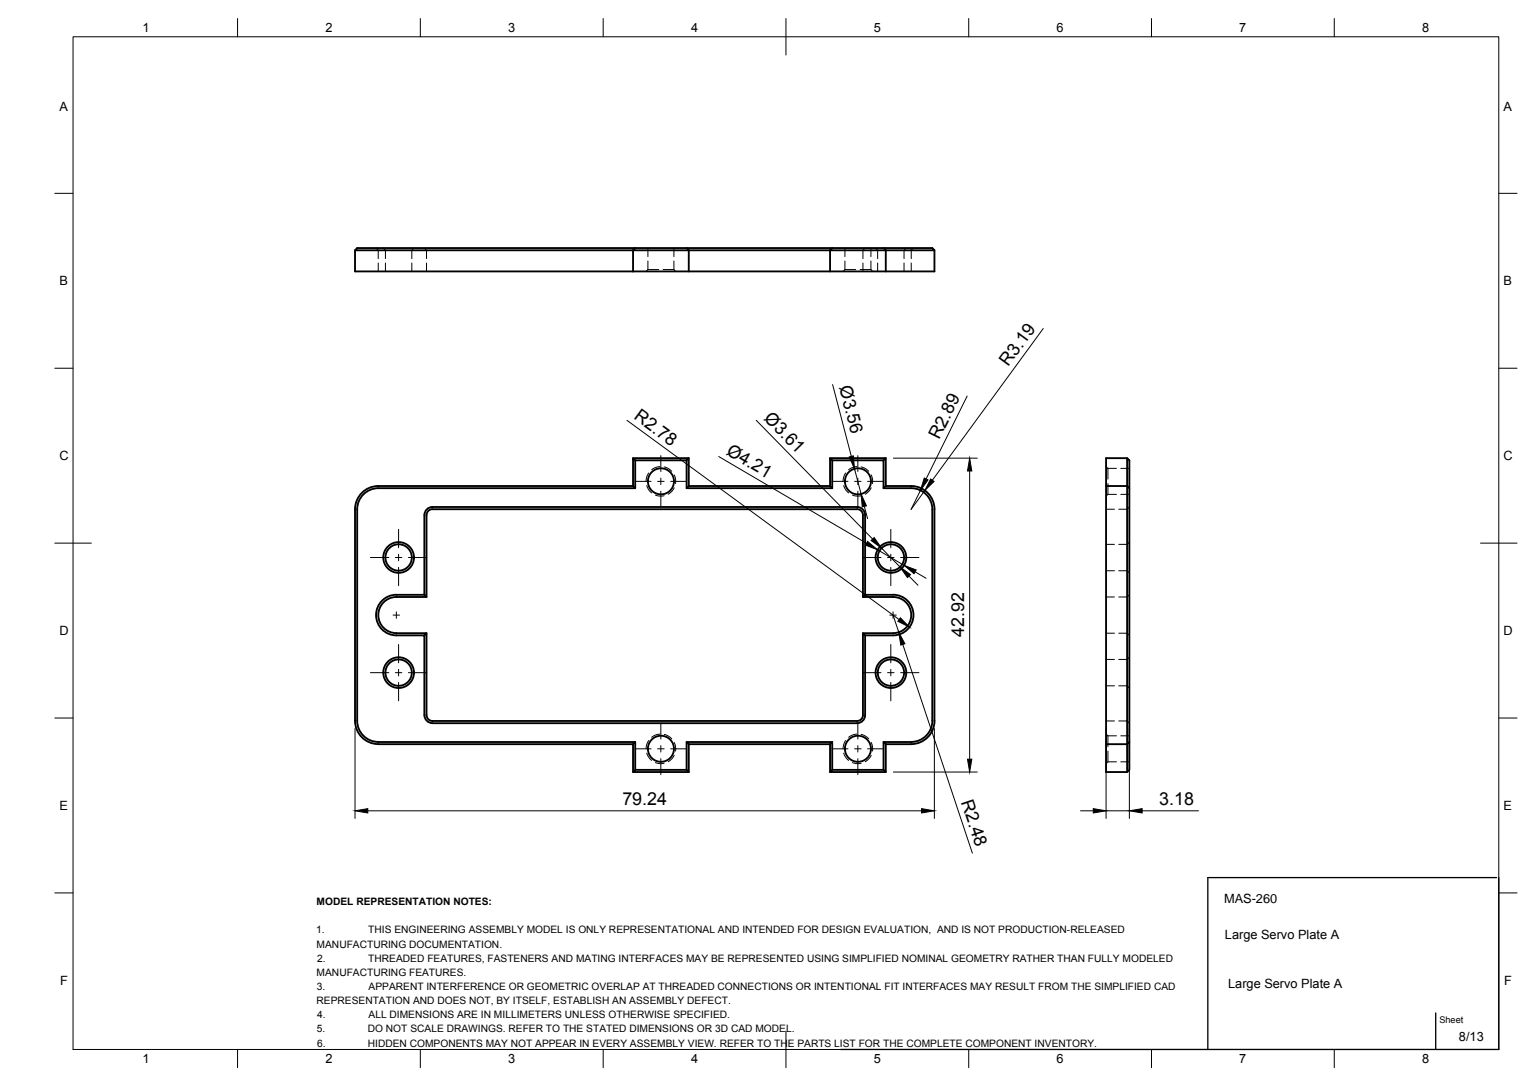
ISO-10303-21;
HEADER;
/* Generated by software containing ST-Developer
 * from STEP Tools, Inc. (www.steptools.com) 
 */

FILE_DESCRIPTION(
/* description */ (''),
/* implementation_level */ '2;1');

FILE_NAME(
/* name */ 'Large Servo Plate A.step',
/* time_stamp */ '2026-10-15T13:29:10-07:00',
/* author */ (''),
/* organization */ (''),
/* preprocessor_version */ 'ST-DEVELOPER v20.2',
/* originating_system */ 'Autodesk Translation Framework v15.15.0.0',
/* authorisation */ '');

FILE_SCHEMA (('AUTOMOTIVE_DESIGN { 1 0 10303 214 3 1 1 }'));
ENDSEC;

DATA;
#10=MECHANICAL_DESIGN_GEOMETRIC_PRESENTATION_REPRESENTATION('',(#934),#83219);
#906=SHAPE_REPRESENTATION_RELATIONSHIP('SRR','None',#83301,#920);
#920=ADVANCED_BREP_SHAPE_REPRESENTATION('',(#948),#83206);
#934=STYLED_ITEM('',(#83380),#948);
#948=MANIFOLD_SOLID_BREP('Body1',#26930);
#983=FACE_BOUND('',#3828,.T.);
#984=FACE_BOUND('',#3829,.T.);
#985=FACE_BOUND('',#3830,.T.);
#986=FACE_BOUND('',#3831,.T.);
#987=FACE_BOUND('',#3832,.T.);
#988=FACE_BOUND('',#3833,.T.);
#989=FACE_BOUND('',#3834,.T.);
#990=FACE_BOUND('',#3835,.T.);
#991=FACE_BOUND('',#3836,.T.);
#992=FACE_BOUND('',#3846,.T.);
#993=FACE_BOUND('',#3847,.T.);
#994=FACE_BOUND('',#3848,.T.);
#995=FACE_BOUND('',#3849,.T.);
#996=FACE_BOUND('',#3850,.T.);
#997=FACE_BOUND('',#3851,.T.);
#998=FACE_BOUND('',#3852,.T.);
#999=FACE_BOUND('',#3853,.T.);
#1000=FACE_BOUND('',#3854,.T.);
#1165=PLANE('',#27211);
#1166=PLANE('',#27246);
#1167=PLANE('',#27270);
#1168=PLANE('',#27271);
#1169=PLANE('',#27272);
#1170=PLANE('',#27273);
#1171=PLANE('',#27274);
#1172=PLANE('',#27275);
#1173=PLANE('',#27276);
#1174=PLANE('',#27277);
#1175=PLANE('',#27278);
#1176=PLANE('',#27279);
#1177=PLANE('',#27280);
#1178=PLANE('',#27281);
#1179=PLANE('',#27282);
#1180=PLANE('',#27285);
#1181=PLANE('',#27288);
#1182=PLANE('',#27291);
#1183=PLANE('',#27294);
#1184=PLANE('',#27295);
#1185=PLANE('',#27296);
#1186=PLANE('',#27297);
#1187=PLANE('',#27298);
#1188=PLANE('',#27299);
#1189=PLANE('',#27300);
#1190=PLANE('',#27301);
#1191=PLANE('',#27302);
#1192=PLANE('',#27303);
#1193=PLANE('',#27304);
#1194=PLANE('',#27305);
#1195=PLANE('',#27307);
#1196=PLANE('',#27309);
#1197=PLANE('',#27310);
#1198=PLANE('',#27311);
#1199=PLANE('',#27312);
#1200=PLANE('',#27315);
#1201=PLANE('',#27316);
#1202=PLANE('',#27319);
#1203=PLANE('',#27322);
#1204=PLANE('',#27325);
#1205=PLANE('',#27328);
#1206=PLANE('',#27331);
#1207=PLANE('',#27332);
#1208=PLANE('',#27334);
#1209=PLANE('',#27335);
#1210=PLANE('',#27337);
#1211=PLANE('',#27339);
#1212=PLANE('',#27340);
#1213=PLANE('',#27341);
#1214=PLANE('',#27343);
#1215=PLANE('',#27344);
#1216=PLANE('',#27346);
#1217=PLANE('',#27348);
#1218=PLANE('',#27349);
#1219=PLANE('',#27350);
#1220=PLANE('',#27351);
#1221=PLANE('',#27352);
#1222=PLANE('',#27353);
#1223=PLANE('',#27354);
#1224=PLANE('',#27355);
#1225=PLANE('',#27357);
#1226=PLANE('',#27359);
#2155=CYLINDRICAL_SURFACE('',#27229,1.778);
#2156=CYLINDRICAL_SURFACE('',#27233,1.778);
#2157=CYLINDRICAL_SURFACE('',#27237,1.778);
#2158=CYLINDRICAL_SURFACE('',#27241,1.778);
#2159=CYLINDRICAL_SURFACE('',#27260,1.8025);
#2160=CYLINDRICAL_SURFACE('',#27263,1.8025);
#2161=CYLINDRICAL_SURFACE('',#27266,1.8025);
#2162=CYLINDRICAL_SURFACE('',#27269,1.8025);
#2163=CYLINDRICAL_SURFACE('',#27306,3.19);
#2164=CYLINDRICAL_SURFACE('',#27308,3.19);
#2165=CYLINDRICAL_SURFACE('',#27333,2.475);
#2166=CYLINDRICAL_SURFACE('',#27336,0.799999999999992);
#2167=CYLINDRICAL_SURFACE('',#27338,0.799999999999994);
#2168=CYLINDRICAL_SURFACE('',#27342,2.475);
#2169=CYLINDRICAL_SURFACE('',#27345,0.799999999999994);
#2170=CYLINDRICAL_SURFACE('',#27347,0.799999999999994);
#2171=CYLINDRICAL_SURFACE('',#27356,3.19);
#2172=CYLINDRICAL_SURFACE('',#27358,3.19);
#2425=FACE_OUTER_BOUND('',#3826,.T.);
#2426=FACE_OUTER_BOUND('',#3827,.T.);
#2427=FACE_OUTER_BOUND('',#3837,.T.);
#2428=FACE_OUTER_BOUND('',#3838,.T.);
#2429=FACE_OUTER_BOUND('',#3839,.T.);
#2430=FACE_OUTER_BOUND('',#3840,.T.);
#2431=FACE_OUTER_BOUND('',#3841,.T.);
#2432=FACE_OUTER_BOUND('',#3842,.T.);
#2433=FACE_OUTER_BOUND('',#3843,.T.);
#2434=FACE_OUTER_BOUND('',#3844,.T.);
#2435=FACE_OUTER_BOUND('',#3845,.T.);
#2436=FACE_OUTER_BOUND('',#3855,.T.);
#2437=FACE_OUTER_BOUND('',#3856,.T.);
#2438=FACE_OUTER_BOUND('',#3857,.T.);
#2439=FACE_OUTER_BOUND('',#3858,.T.);
#2440=FACE_OUTER_BOUND('',#3859,.T.);
#2441=FACE_OUTER_BOUND('',#3860,.T.);
#2442=FACE_OUTER_BOUND('',#3861,.T.);
#2443=FACE_OUTER_BOUND('',#3862,.T.);
#2444=FACE_OUTER_BOUND('',#3863,.T.);
#2445=FACE_OUTER_BOUND('',#3864,.T.);
#2446=FACE_OUTER_BOUND('',#3865,.T.);
#2447=FACE_OUTER_BOUND('',#3866,.T.);
#2448=FACE_OUTER_BOUND('',#3867,.T.);
#2449=FACE_OUTER_BOUND('',#3868,.T.);
#2450=FACE_OUTER_BOUND('',#3869,.T.);
#2451=FACE_OUTER_BOUND('',#3870,.T.);
#2452=FACE_OUTER_BOUND('',#3871,.T.);
#2453=FACE_OUTER_BOUND('',#3872,.T.);
#2454=FACE_OUTER_BOUND('',#3873,.T.);
#2455=FACE_OUTER_BOUND('',#3874,.T.);
#2456=FACE_OUTER_BOUND('',#3875,.T.);
#2457=FACE_OUTER_BOUND('',#3876,.T.);
#2458=FACE_OUTER_BOUND('',#3877,.T.);
#2459=FACE_OUTER_BOUND('',#3878,.T.);
#2460=FACE_OUTER_BOUND('',#3879,.T.);
#2461=FACE_OUTER_BOUND('',#3880,.T.);
#2462=FACE_OUTER_BOUND('',#3881,.T.);
#2463=FACE_OUTER_BOUND('',#3882,.T.);
#2464=FACE_OUTER_BOUND('',#3883,.T.);
#2465=FACE_OUTER_BOUND('',#3884,.T.);
#2466=FACE_OUTER_BOUND('',#3885,.T.);
#2467=FACE_OUTER_BOUND('',#3886,.T.);
#2468=FACE_OUTER_BOUND('',#3887,.T.);
#2469=FACE_OUTER_BOUND('',#3888,.T.);
#2470=FACE_OUTER_BOUND('',#3889,.T.);
#2471=FACE_OUTER_BOUND('',#3890,.T.);
#2472=FACE_OUTER_BOUND('',#3891,.T.);
#2473=FACE_OUTER_BOUND('',#3892,.T.);
#2474=FACE_OUTER_BOUND('',#3893,.T.);
#2475=FACE_OUTER_BOUND('',#3894,.T.);
#2476=FACE_OUTER_BOUND('',#3895,.T.);
#2477=FACE_OUTER_BOUND('',#3896,.T.);
#2478=FACE_OUTER_BOUND('',#3897,.T.);
#2479=FACE_OUTER_BOUND('',#3898,.T.);
#2480=FACE_OUTER_BOUND('',#3899,.T.);
#2481=FACE_OUTER_BOUND('',#3900,.T.);
#2482=FACE_OUTER_BOUND('',#3901,.T.);
#2483=FACE_OUTER_BOUND('',#3902,.T.);
#2484=FACE_OUTER_BOUND('',#3903,.T.);
#2485=FACE_OUTER_BOUND('',#3904,.T.);
#2486=FACE_OUTER_BOUND('',#3905,.T.);
#2487=FACE_OUTER_BOUND('',#3906,.T.);
#2488=FACE_OUTER_BOUND('',#3907,.T.);
#2489=FACE_OUTER_BOUND('',#3908,.T.);
#2490=FACE_OUTER_BOUND('',#3909,.T.);
#2491=FACE_OUTER_BOUND('',#3910,.T.);
#2492=FACE_OUTER_BOUND('',#3911,.T.);
#2493=FACE_OUTER_BOUND('',#3912,.T.);
#2494=FACE_OUTER_BOUND('',#3913,.T.);
#2495=FACE_OUTER_BOUND('',#3914,.T.);
#2496=FACE_OUTER_BOUND('',#3915,.T.);
#2497=FACE_OUTER_BOUND('',#3916,.T.);
#2498=FACE_OUTER_BOUND('',#3917,.T.);
#2499=FACE_OUTER_BOUND('',#3918,.T.);
#2500=FACE_OUTER_BOUND('',#3919,.T.);
#2501=FACE_OUTER_BOUND('',#3920,.T.);
#2502=FACE_OUTER_BOUND('',#3921,.T.);
#2503=FACE_OUTER_BOUND('',#3922,.T.);
#2504=FACE_OUTER_BOUND('',#3923,.T.);
#2505=FACE_OUTER_BOUND('',#3924,.T.);
#2506=FACE_OUTER_BOUND('',#3925,.T.);
#2507=FACE_OUTER_BOUND('',#3926,.T.);
#2508=FACE_OUTER_BOUND('',#3927,.T.);
#2509=FACE_OUTER_BOUND('',#3928,.T.);
#2510=FACE_OUTER_BOUND('',#3929,.T.);
#2511=FACE_OUTER_BOUND('',#3930,.T.);
#2512=FACE_OUTER_BOUND('',#3931,.T.);
#2513=FACE_OUTER_BOUND('',#3932,.T.);
#2514=FACE_OUTER_BOUND('',#3933,.T.);
#2515=FACE_OUTER_BOUND('',#3934,.T.);
#2516=FACE_OUTER_BOUND('',#3935,.T.);
#2517=FACE_OUTER_BOUND('',#3936,.T.);
#2518=FACE_OUTER_BOUND('',#3937,.T.);
#2519=FACE_OUTER_BOUND('',#3938,.T.);
#2520=FACE_OUTER_BOUND('',#3939,.T.);
#2521=FACE_OUTER_BOUND('',#3940,.T.);
#2522=FACE_OUTER_BOUND('',#3941,.T.);
#3826=EDGE_LOOP('',(#17916,#17917,#17918,#17919));
#3827=EDGE_LOOP('',(#17920,#17921,#17922,#17923,#17924,#17925,#17926,#17927,
#17928,#17929,#17930,#17931,#17932,#17933,#17934,#17935,#17936,#17937,#17938,
#17939,#17940,#17941,#17942,#17943));
#3828=EDGE_LOOP('',(#17944));
#3829=EDGE_LOOP('',(#17945));
#3830=EDGE_LOOP('',(#17946));
#3831=EDGE_LOOP('',(#17947));
#3832=EDGE_LOOP('',(#17948));
#3833=EDGE_LOOP('',(#17949));
#3834=EDGE_LOOP('',(#17950,#17951,#17952,#17953,#17954,#17955,#17956,#17957,
#17958,#17959,#17960,#17961,#17962,#17963,#17964,#17965));
#3835=EDGE_LOOP('',(#17966));
#3836=EDGE_LOOP('',(#17967));
#3837=EDGE_LOOP('',(#17968,#17969,#17970,#17971));
#3838=EDGE_LOOP('',(#17972,#17973,#17974,#17975));
#3839=EDGE_LOOP('',(#17976,#17977,#17978,#17979));
#3840=EDGE_LOOP('',(#17980,#17981,#17982,#17983));
#3841=EDGE_LOOP('',(#17984,#17985,#17986,#17987));
#3842=EDGE_LOOP('',(#17988,#17989,#17990,#17991));
#3843=EDGE_LOOP('',(#17992,#17993,#17994,#17995));
#3844=EDGE_LOOP('',(#17996,#17997,#17998,#17999));
#3845=EDGE_LOOP('',(#18000,#18001,#18002,#18003,#18004,#18005,#18006,#18007,
#18008,#18009,#18010,#18011,#18012,#18013,#18014,#18015,#18016,#18017,#18018,
#18019,#18020,#18021,#18022,#18023));
#3846=EDGE_LOOP('',(#18024));
#3847=EDGE_LOOP('',(#18025));
#3848=EDGE_LOOP('',(#18026,#18027,#18028,#18029,#18030,#18031,#18032,#18033,
#18034,#18035,#18036,#18037,#18038,#18039,#18040,#18041));
#3849=EDGE_LOOP('',(#18042));
#3850=EDGE_LOOP('',(#18043));
#3851=EDGE_LOOP('',(#18044));
#3852=EDGE_LOOP('',(#18045));
#3853=EDGE_LOOP('',(#18046));
#3854=EDGE_LOOP('',(#18047));
#3855=EDGE_LOOP('',(#18048,#18049,#18050,#18051));
#3856=EDGE_LOOP('',(#18052,#18053,#18054,#18055));
#3857=EDGE_LOOP('',(#18056,#18057,#18058,#18059));
#3858=EDGE_LOOP('',(#18060,#18061,#18062,#18063));
#3859=EDGE_LOOP('',(#18064,#18065,#18066,#18067));
#3860=EDGE_LOOP('',(#18068,#18069,#18070,#18071));
#3861=EDGE_LOOP('',(#18072,#18073,#18074,#18075));
#3862=EDGE_LOOP('',(#18076,#18077,#18078,#18079));
#3863=EDGE_LOOP('',(#18080,#18081,#18082,#18083));
#3864=EDGE_LOOP('',(#18084,#18085,#18086,#18087));
#3865=EDGE_LOOP('',(#18088,#18089,#18090,#18091));
#3866=EDGE_LOOP('',(#18092,#18093,#18094,#18095));
#3867=EDGE_LOOP('',(#18096,#18097,#18098,#18099));
#3868=EDGE_LOOP('',(#18100,#18101,#18102,#18103));
#3869=EDGE_LOOP('',(#18104,#18105,#18106,#18107));
#3870=EDGE_LOOP('',(#18108,#18109,#18110,#18111));
#3871=EDGE_LOOP('',(#18112,#18113,#18114,#18115));
#3872=EDGE_LOOP('',(#18116,#18117,#18118,#18119));
#3873=EDGE_LOOP('',(#18120,#18121,#18122,#18123));
#3874=EDGE_LOOP('',(#18124,#18125,#18126,#18127));
#3875=EDGE_LOOP('',(#18128,#18129,#18130,#18131));
#3876=EDGE_LOOP('',(#18132,#18133,#18134,#18135));
#3877=EDGE_LOOP('',(#18136,#18137,#18138,#18139));
#3878=EDGE_LOOP('',(#18140,#18141,#18142,#18143));
#3879=EDGE_LOOP('',(#18144,#18145,#18146,#18147));
#3880=EDGE_LOOP('',(#18148,#18149,#18150,#18151));
#3881=EDGE_LOOP('',(#18152,#18153,#18154,#18155));
#3882=EDGE_LOOP('',(#18156,#18157,#18158,#18159));
#3883=EDGE_LOOP('',(#18160,#18161,#18162,#18163));
#3884=EDGE_LOOP('',(#18164,#18165,#18166,#18167));
#3885=EDGE_LOOP('',(#18168,#18169,#18170,#18171));
#3886=EDGE_LOOP('',(#18172,#18173,#18174,#18175));
#3887=EDGE_LOOP('',(#18176,#18177,#18178,#18179));
#3888=EDGE_LOOP('',(#18180,#18181,#18182,#18183));
#3889=EDGE_LOOP('',(#18184,#18185,#18186,#18187));
#3890=EDGE_LOOP('',(#18188,#18189,#18190,#18191));
#3891=EDGE_LOOP('',(#18192,#18193,#18194,#18195));
#3892=EDGE_LOOP('',(#18196,#18197,#18198,#18199));
#3893=EDGE_LOOP('',(#18200,#18201,#18202,#18203));
#3894=EDGE_LOOP('',(#18204,#18205,#18206,#18207));
#3895=EDGE_LOOP('',(#18208,#18209,#18210,#18211));
#3896=EDGE_LOOP('',(#18212,#18213,#18214,#18215));
#3897=EDGE_LOOP('',(#18216,#18217,#18218,#18219));
#3898=EDGE_LOOP('',(#18220,#18221,#18222,#18223));
#3899=EDGE_LOOP('',(#18224,#18225,#18226,#18227));
#3900=EDGE_LOOP('',(#18228,#18229,#18230,#18231));
#3901=EDGE_LOOP('',(#18232,#18233,#18234,#18235));
#3902=EDGE_LOOP('',(#18236,#18237,#18238,#18239));
#3903=EDGE_LOOP('',(#18240,#18241,#18242,#18243));
#3904=EDGE_LOOP('',(#18244,#18245,#18246,#18247));
#3905=EDGE_LOOP('',(#18248,#18249,#18250,#18251));
#3906=EDGE_LOOP('',(#18252,#18253,#18254,#18255));
#3907=EDGE_LOOP('',(#18256,#18257,#18258,#18259));
#3908=EDGE_LOOP('',(#18260,#18261,#18262,#18263));
#3909=EDGE_LOOP('',(#18264,#18265,#18266,#18267));
#3910=EDGE_LOOP('',(#18268,#18269,#18270,#18271));
#3911=EDGE_LOOP('',(#18272,#18273,#18274,#18275));
#3912=EDGE_LOOP('',(#18276,#18277,#18278,#18279));
#3913=EDGE_LOOP('',(#18280,#18281,#18282,#18283));
#3914=EDGE_LOOP('',(#18284,#18285,#18286,#18287));
#3915=EDGE_LOOP('',(#18288,#18289,#18290,#18291));
#3916=EDGE_LOOP('',(#18292,#18293,#18294,#18295));
#3917=EDGE_LOOP('',(#18296,#18297,#18298,#18299));
#3918=EDGE_LOOP('',(#18300,#18301,#18302,#18303));
#3919=EDGE_LOOP('',(#18304,#18305,#18306,#18307));
#3920=EDGE_LOOP('',(#18308,#18309,#18310,#18311));
#3921=EDGE_LOOP('',(#18312,#18313,#18314,#18315));
#3922=EDGE_LOOP('',(#18316,#18317,#18318,#18319));
#3923=EDGE_LOOP('',(#18320,#18321,#18322,#18323));
#3924=EDGE_LOOP('',(#18324,#18325,#18326,#18327));
#3925=EDGE_LOOP('',(#18328,#18329,#18330,#18331));
#3926=EDGE_LOOP('',(#18332,#18333,#18334,#18335));
#3927=EDGE_LOOP('',(#18336,#18337,#18338,#18339));
#3928=EDGE_LOOP('',(#18340,#18341,#18342,#18343));
#3929=EDGE_LOOP('',(#18344,#18345,#18346,#18347));
#3930=EDGE_LOOP('',(#18348,#18349,#18350,#18351));
#3931=EDGE_LOOP('',(#18352,#18353,#18354,#18355));
#3932=EDGE_LOOP('',(#18356,#18357,#18358,#18359));
#3933=EDGE_LOOP('',(#18360,#18361,#18362,#18363));
#3934=EDGE_LOOP('',(#18364,#18365,#18366,#18367));
#3935=EDGE_LOOP('',(#18368,#18369,#18370,#18371));
#3936=EDGE_LOOP('',(#18372,#18373,#18374,#18375));
#3937=EDGE_LOOP('',(#18376,#18377,#18378,#18379));
#3938=EDGE_LOOP('',(#18380,#18381,#18382,#18383));
#3939=EDGE_LOOP('',(#18384,#18385,#18386,#18387));
#3940=EDGE_LOOP('',(#18388,#18389,#18390,#18391));
#3941=EDGE_LOOP('',(#18392,#18393,#18394,#18395));
#5403=LINE('',#36423,#7914);
#5404=LINE('',#36428,#7915);
#5405=LINE('',#36432,#7916);
#5406=LINE('',#36436,#7917);
#5407=LINE('',#36438,#7918);
#5408=LINE('',#36440,#7919);
#5409=LINE('',#36442,#7920);
#5410=LINE('',#36444,#7921);
#5411=LINE('',#36446,#7922);
#5412=LINE('',#36448,#7923);
#5413=LINE('',#36450,#7924);
#5414=LINE('',#36452,#7925);
#5415=LINE('',#36456,#7926);
#5416=LINE('',#36460,#7927);
#5417=LINE('',#36462,#7928);
#5418=LINE('',#36464,#7929);
#5419=LINE('',#36466,#7930);
#5420=LINE('',#36468,#7931);
#5421=LINE('',#36470,#7932);
#5422=LINE('',#36472,#7933);
#5423=LINE('',#36473,#7934);
#5424=LINE('',#36488,#7935);
#5425=LINE('',#36490,#7936);
#5426=LINE('',#36494,#7937);
#5427=LINE('',#36498,#7938);
#5428=LINE('',#36500,#7939);
#5429=LINE('',#36504,#7940);
#5430=LINE('',#36506,#7941);
#5431=LINE('',#36510,#7942);
#5432=LINE('',#36514,#7943);
#5433=LINE('',#36516,#7944);
#5434=LINE('',#36523,#7945);
#5435=LINE('',#36527,#7946);
#5436=LINE('',#36531,#7947);
#5437=LINE('',#36535,#7948);
#5438=LINE('',#36539,#7949);
#5439=LINE('',#36543,#7950);
#5440=LINE('',#36547,#7951);
#5441=LINE('',#36552,#7952);
#5442=LINE('',#36557,#7953);
#5443=LINE('',#36561,#7954);
#5444=LINE('',#36565,#7955);
#5445=LINE('',#36567,#7956);
#5446=LINE('',#36569,#7957);
#5447=LINE('',#36571,#7958);
#5448=LINE('',#36573,#7959);
#5449=LINE('',#36575,#7960);
#5450=LINE('',#36577,#7961);
#5451=LINE('',#36579,#7962);
#5452=LINE('',#36581,#7963);
#5453=LINE('',#36585,#7964);
#5454=LINE('',#36589,#7965);
#5455=LINE('',#36591,#7966);
#5456=LINE('',#36593,#7967);
#5457=LINE('',#36595,#7968);
#5458=LINE('',#36597,#7969);
#5459=LINE('',#36599,#7970);
#5460=LINE('',#36601,#7971);
#5461=LINE('',#36602,#7972);
#5462=LINE('',#36607,#7973);
#5463=LINE('',#36611,#7974);
#5464=LINE('',#36615,#7975);
#5465=LINE('',#36617,#7976);
#5466=LINE('',#36621,#7977);
#5467=LINE('',#36623,#7978);
#5468=LINE('',#36627,#7979);
#5469=LINE('',#36631,#7980);
#5470=LINE('',#36633,#7981);
#5471=LINE('',#36636,#7982);
#5472=LINE('',#36642,#7983);
#5473=LINE('',#36646,#7984);
#5474=LINE('',#36648,#7985);
#5475=LINE('',#36652,#7986);
#5476=LINE('',#36654,#7987);
#5477=LINE('',#36658,#7988);
#5478=LINE('',#36660,#7989);
#5479=LINE('',#36663,#7990);
#5480=LINE('',#36665,#7991);
#5481=LINE('',#36666,#7992);
#5482=LINE('',#36669,#7993);
#5483=LINE('',#36670,#7994);
#5484=LINE('',#36673,#7995);
#5485=LINE('',#36674,#7996);
#5486=LINE('',#36677,#7997);
#5487=LINE('',#36678,#7998);
#5488=LINE('',#36682,#7999);
#5489=LINE('',#36683,#8000);
#5490=LINE('',#36684,#8001);
#5491=LINE('',#36687,#8002);
#5492=LINE('',#36688,#8003);
#5493=LINE('',#36691,#8004);
#5494=LINE('',#36692,#8005);
#5495=LINE('',#36695,#8006);
#5496=LINE('',#36696,#8007);
#5497=LINE('',#36699,#8008);
#5498=LINE('',#36700,#8009);
#5499=LINE('',#36703,#8010);
#5500=LINE('',#36704,#8011);
#5501=LINE('',#36707,#8012);
#5502=LINE('',#36708,#8013);
#5503=LINE('',#36711,#8014);
#5504=LINE('',#36712,#8015);
#5505=LINE('',#36716,#8016);
#5506=LINE('',#36717,#8017);
#5507=LINE('',#36718,#8018);
#5508=LINE('',#36721,#8019);
#5509=LINE('',#36725,#8020);
#5510=LINE('',#36726,#8021);
#5511=LINE('',#36729,#8022);
#5512=LINE('',#36732,#8023);
#5513=LINE('',#36735,#8024);
#5514=LINE('',#36739,#8025);
#5515=LINE('',#36740,#8026);
#5516=LINE('',#36743,#8027);
#5517=LINE('',#36746,#8028);
#5518=LINE('',#36749,#8029);
#5519=LINE('',#36750,#8030);
#5520=LINE('',#36753,#8031);
#5521=LINE('',#36754,#8032);
#5522=LINE('',#36756,#8033);
#5523=LINE('',#36758,#8034);
#5524=LINE('',#36759,#8035);
#5525=LINE('',#36761,#8036);
#5526=LINE('',#36763,#8037);
#5527=LINE('',#36765,#8038);
#5528=LINE('',#36767,#8039);
#5529=LINE('',#36769,#8040);
#5530=LINE('',#36771,#8041);
#5531=LINE('',#36773,#8042);
#5532=LINE('',#36775,#8043);
#5533=LINE('',#36777,#8044);
#5534=LINE('',#36779,#8045);
#5535=LINE('',#36781,#8046);
#5536=LINE('',#36785,#8047);
#5537=LINE('',#36786,#8048);
#5538=LINE('',#36787,#8049);
#5539=LINE('',#36791,#8050);
#5540=LINE('',#36792,#8051);
#5541=LINE('',#36793,#8052);
#5542=LINE('',#36797,#8053);
#5543=LINE('',#36798,#8054);
#5544=LINE('',#36799,#8055);
#5545=LINE('',#36802,#8056);
#5546=LINE('',#36805,#8057);
#5547=LINE('',#36809,#8058);
#5548=LINE('',#36810,#8059);
#5549=LINE('',#36811,#8060);
#5550=LINE('',#36814,#8061);
#5551=LINE('',#36818,#8062);
#5552=LINE('',#36819,#8063);
#5553=LINE('',#36822,#8064);
#5554=LINE('',#36825,#8065);
#5555=LINE('',#36828,#8066);
#5556=LINE('',#36832,#8067);
#5557=LINE('',#36833,#8068);
#5558=LINE('',#36836,#8069);
#5559=LINE('',#36839,#8070);
#5560=LINE('',#36842,#8071);
#5561=LINE('',#36845,#8072);
#5562=LINE('',#36847,#8073);
#5563=LINE('',#36848,#8074);
#5564=LINE('',#36850,#8075);
#5565=LINE('',#36852,#8076);
#5566=LINE('',#36854,#8077);
#5567=LINE('',#36856,#8078);
#5568=LINE('',#36858,#8079);
#5569=LINE('',#36860,#8080);
#5570=LINE('',#36862,#8081);
#5571=LINE('',#36864,#8082);
#5572=LINE('',#36866,#8083);
#5573=LINE('',#36867,#8084);
#5574=LINE('',#36870,#8085);
#5575=LINE('',#36872,#8086);
#5576=LINE('',#36874,#8087);
#5577=LINE('',#36876,#8088);
#5578=LINE('',#36879,#8089);
#5579=LINE('',#36881,#8090);
#5580=LINE('',#36882,#8091);
#5581=LINE('',#36885,#8092);
#5582=LINE('',#36887,#8093);
#5583=LINE('',#36888,#8094);
#5584=LINE('',#36890,#8095);
#5585=LINE('',#36893,#8096);
#5586=LINE('',#36895,#8097);
#5587=LINE('',#36897,#8098);
#5588=LINE('',#36899,#8099);
#7914=VECTOR('',#29605,1.903);
#7915=VECTOR('',#29610,10.);
#7916=VECTOR('',#29613,10.);
#7917=VECTOR('',#29616,10.);
#7918=VECTOR('',#29617,10.);
#7919=VECTOR('',#29618,10.);
#7920=VECTOR('',#29619,10.);
#7921=VECTOR('',#29620,10.);
#7922=VECTOR('',#29621,10.);
#7923=VECTOR('',#29622,10.);
#7924=VECTOR('',#29623,10.);
#7925=VECTOR('',#29624,10.);
#7926=VECTOR('',#29627,10.);
#7927=VECTOR('',#29630,10.);
#7928=VECTOR('',#29631,10.);
#7929=VECTOR('',#29632,10.);
#7930=VECTOR('',#29633,10.);
#7931=VECTOR('',#29634,10.);
#7932=VECTOR('',#29635,10.);
#7933=VECTOR('',#29636,10.);
#7934=VECTOR('',#29637,10.);
#7935=VECTOR('',#29650,10.);
#7936=VECTOR('',#29651,10.);
#7937=VECTOR('',#29654,10.);
#7938=VECTOR('',#29657,10.);
#7939=VECTOR('',#29658,10.);
#7940=VECTOR('',#29661,10.);
#7941=VECTOR('',#29662,10.);
#7942=VECTOR('',#29665,10.);
#7943=VECTOR('',#29668,10.);
#7944=VECTOR('',#29669,10.);
#7945=VECTOR('',#29678,1.778);
#7946=VECTOR('',#29683,1.903);
#7947=VECTOR('',#29688,1.778);
#7948=VECTOR('',#29693,1.903);
#7949=VECTOR('',#29698,1.778);
#7950=VECTOR('',#29703,1.903);
#7951=VECTOR('',#29708,1.778);
#7952=VECTOR('',#29713,1.9525);
#7953=VECTOR('',#29718,10.);
#7954=VECTOR('',#29721,10.);
#7955=VECTOR('',#29724,10.);
#7956=VECTOR('',#29725,10.);
#7957=VECTOR('',#29726,10.);
#7958=VECTOR('',#29727,10.);
#7959=VECTOR('',#29728,10.);
#7960=VECTOR('',#29729,10.);
#7961=VECTOR('',#29730,10.);
#7962=VECTOR('',#29731,10.);
#7963=VECTOR('',#29732,10.);
#7964=VECTOR('',#29735,10.);
#7965=VECTOR('',#29738,10.);
#7966=VECTOR('',#29739,10.);
#7967=VECTOR('',#29740,10.);
#7968=VECTOR('',#29741,10.);
#7969=VECTOR('',#29742,10.);
#7970=VECTOR('',#29743,10.);
#7971=VECTOR('',#29744,10.);
#7972=VECTOR('',#29745,10.);
#7973=VECTOR('',#29748,10.);
#7974=VECTOR('',#29751,10.);
#7975=VECTOR('',#29754,10.);
#7976=VECTOR('',#29755,10.);
#7977=VECTOR('',#29758,10.);
#7978=VECTOR('',#29759,10.);
#7979=VECTOR('',#29762,10.);
#7980=VECTOR('',#29765,10.);
#7981=VECTOR('',#29766,10.);
#7982=VECTOR('',#29769,10.);
#7983=VECTOR('',#29776,1.8025);
#7984=VECTOR('',#29781,1.9525);
#7985=VECTOR('',#29784,1.8025);
#7986=VECTOR('',#29789,1.9525);
#7987=VECTOR('',#29792,1.8025);
#7988=VECTOR('',#29797,1.9525);
#7989=VECTOR('',#29800,1.8025);
#7990=VECTOR('',#29803,10.);
#7991=VECTOR('',#29804,10.);
#7992=VECTOR('',#29805,10.);
#7993=VECTOR('',#29808,10.);
#7994=VECTOR('',#29809,10.);
#7995=VECTOR('',#29812,10.);
#7996=VECTOR('',#29813,10.);
#7997=VECTOR('',#29816,10.);
#7998=VECTOR('',#29817,10.);
#7999=VECTOR('',#29820,10.);
#8000=VECTOR('',#29821,10.);
#8001=VECTOR('',#29822,10.);
#8002=VECTOR('',#29825,10.);
#8003=VECTOR('',#29826,10.);
#8004=VECTOR('',#29829,10.);
#8005=VECTOR('',#29830,10.);
#8006=VECTOR('',#29833,10.);
#8007=VECTOR('',#29834,10.);
#8008=VECTOR('',#29837,10.);
#8009=VECTOR('',#29838,10.);
#8010=VECTOR('',#29841,10.);
#8011=VECTOR('',#29842,10.);
#8012=VECTOR('',#29845,10.);
#8013=VECTOR('',#29846,10.);
#8014=VECTOR('',#29849,10.);
#8015=VECTOR('',#29850,10.);
#8016=VECTOR('',#29853,10.);
#8017=VECTOR('',#29854,10.);
#8018=VECTOR('',#29855,10.);
#8019=VECTOR('',#29858,10.);
#8020=VECTOR('',#29863,10.);
#8021=VECTOR('',#29864,10.);
#8022=VECTOR('',#29867,10.);
#8023=VECTOR('',#29872,10.);
#8024=VECTOR('',#29875,9.99999999999999);
#8025=VECTOR('',#29880,9.99999999999999);
#8026=VECTOR('',#29881,10.);
#8027=VECTOR('',#29884,9.99999999999999);
#8028=VECTOR('',#29889,10.);
#8029=VECTOR('',#29892,10.);
#8030=VECTOR('',#29893,10.);
#8031=VECTOR('',#29896,10.);
#8032=VECTOR('',#29897,10.);
#8033=VECTOR('',#29900,10.);
#8034=VECTOR('',#29903,10.);
#8035=VECTOR('',#29904,10.);
#8036=VECTOR('',#29907,10.);
#8037=VECTOR('',#29910,10.);
#8038=VECTOR('',#29913,10.);
#8039=VECTOR('',#29916,10.);
#8040=VECTOR('',#29919,10.);
#8041=VECTOR('',#29922,10.);
#8042=VECTOR('',#29925,10.);
#8043=VECTOR('',#29928,10.);
#8044=VECTOR('',#29931,10.);
#8045=VECTOR('',#29934,10.);
#8046=VECTOR('',#29937,10.);
#8047=VECTOR('',#29940,10.);
#8048=VECTOR('',#29941,10.);
#8049=VECTOR('',#29942,10.);
#8050=VECTOR('',#29945,10.);
#8051=VECTOR('',#29946,10.);
#8052=VECTOR('',#29947,10.);
#8053=VECTOR('',#29950,10.);
#8054=VECTOR('',#29951,10.);
#8055=VECTOR('',#29952,10.);
#8056=VECTOR('',#29955,10.);
#8057=VECTOR('',#29960,10.);
#8058=VECTOR('',#29963,10.);
#8059=VECTOR('',#29964,10.);
#8060=VECTOR('',#29965,10.);
#8061=VECTOR('',#29968,10.);
#8062=VECTOR('',#29973,10.);
#8063=VECTOR('',#29974,10.);
#8064=VECTOR('',#29977,10.);
#8065=VECTOR('',#29982,10.);
#8066=VECTOR('',#29985,10.);
#8067=VECTOR('',#29990,10.);
#8068=VECTOR('',#29991,10.);
#8069=VECTOR('',#29994,10.);
#8070=VECTOR('',#29999,10.);
#8071=VECTOR('',#30002,9.99999999999999);
#8072=VECTOR('',#30007,10.);
#8073=VECTOR('',#30010,10.);
#8074=VECTOR('',#30011,10.);
#8075=VECTOR('',#30014,10.);
#8076=VECTOR('',#30017,10.);
#8077=VECTOR('',#30020,10.);
#8078=VECTOR('',#30023,10.);
#8079=VECTOR('',#30026,10.);
#8080=VECTOR('',#30029,10.);
#8081=VECTOR('',#30032,10.);
#8082=VECTOR('',#30035,10.);
#8083=VECTOR('',#30038,10.);
#8084=VECTOR('',#30039,10.);
#8085=VECTOR('',#30044,10.);
#8086=VECTOR('',#30047,10.);
#8087=VECTOR('',#30050,10.);
#8088=VECTOR('',#30053,10.);
#8089=VECTOR('',#30058,10.);
#8090=VECTOR('',#30061,10.);
#8091=VECTOR('',#30062,10.);
#8092=VECTOR('',#30067,10.);
#8093=VECTOR('',#30070,10.);
#8094=VECTOR('',#30071,10.);
#8095=VECTOR('',#30074,10.);
#8096=VECTOR('',#30079,10.);
#8097=VECTOR('',#30082,10.);
#8098=VECTOR('',#30085,10.);
#8099=VECTOR('',#30088,10.);
#10338=CIRCLE('',#27209,1.778);
#10339=CIRCLE('',#27210,2.028);
#10340=CIRCLE('',#27212,3.19);
#10341=CIRCLE('',#27213,3.19);
#10342=CIRCLE('',#27214,3.19);
#10343=CIRCLE('',#27215,3.19);
#10344=CIRCLE('',#27216,2.028);
#10345=CIRCLE('',#27217,2.028);
#10346=CIRCLE('',#27218,1.8025);
#10347=CIRCLE('',#27219,1.8025);
#10348=CIRCLE('',#27220,1.8025);
#10349=CIRCLE('',#27221,1.8025);
#10350=CIRCLE('',#27222,0.799999999999992);
#10351=CIRCLE('',#27223,0.799999999999994);
#10352=CIRCLE('',#27224,2.475);
#10353=CIRCLE('',#27225,0.799999999999994);
#10354=CIRCLE('',#27226,0.799999999999994);
#10355=CIRCLE('',#27227,2.475);
#10356=CIRCLE('',#27228,2.028);
#10357=CIRCLE('',#27230,1.778);
#10358=CIRCLE('',#27232,1.778);
#10359=CIRCLE('',#27234,1.778);
#10360=CIRCLE('',#27236,1.778);
#10361=CIRCLE('',#27238,1.778);
#10362=CIRCLE('',#27240,1.778);
#10363=CIRCLE('',#27242,1.778);
#10364=CIRCLE('',#27244,1.8025);
#10365=CIRCLE('',#27245,2.1025);
#10366=CIRCLE('',#27247,2.89);
#10367=CIRCLE('',#27248,2.88999999999999);
#10368=CIRCLE('',#27249,2.89000000000001);
#10369=CIRCLE('',#27250,2.89);
#10370=CIRCLE('',#27251,2.1025);
#10371=CIRCLE('',#27252,1.09999999999999);
#10372=CIRCLE('',#27253,1.1);
#10373=CIRCLE('',#27254,2.775);
#10374=CIRCLE('',#27255,1.1);
#10375=CIRCLE('',#27256,1.09999999999999);
#10376=CIRCLE('',#27257,2.775);
#10377=CIRCLE('',#27258,2.1025);
#10378=CIRCLE('',#27259,2.1025);
#10379=CIRCLE('',#27262,1.8025);
#10380=CIRCLE('',#27265,1.8025);
#10381=CIRCLE('',#27268,1.8025);
#10382=CIRCLE('',#27284,3.19);
#10383=CIRCLE('',#27287,3.19);
#10384=CIRCLE('',#27290,3.19);
#10385=CIRCLE('',#27293,3.19);
#10386=CIRCLE('',#27314,2.475);
#10387=CIRCLE('',#27318,0.799999999999994);
#10388=CIRCLE('',#27321,0.799999999999992);
#10389=CIRCLE('',#27324,0.799999999999994);
#10390=CIRCLE('',#27327,0.799999999999994);
#10391=CIRCLE('',#27330,2.475);
#11154=VERTEX_POINT('',#36420);
#11155=VERTEX_POINT('',#36422);
#11156=VERTEX_POINT('',#36426);
#11157=VERTEX_POINT('',#36427);
#11158=VERTEX_POINT('',#36429);
#11159=VERTEX_POINT('',#36431);
#11160=VERTEX_POINT('',#36433);
#11161=VERTEX_POINT('',#36435);
#11162=VERTEX_POINT('',#36437);
#11163=VERTEX_POINT('',#36439);
#11164=VERTEX_POINT('',#36441);
#11165=VERTEX_POINT('',#36443);
#11166=VERTEX_POINT('',#36445);
#11167=VERTEX_POINT('',#36447);
#11168=VERTEX_POINT('',#36449);
#11169=VERTEX_POINT('',#36451);
#11170=VERTEX_POINT('',#36453);
#11171=VERTEX_POINT('',#36455);
#11172=VERTEX_POINT('',#36457);
#11173=VERTEX_POINT('',#36459);
#11174=VERTEX_POINT('',#36461);
#11175=VERTEX_POINT('',#36463);
#11176=VERTEX_POINT('',#36465);
#11177=VERTEX_POINT('',#36467);
#11178=VERTEX_POINT('',#36469);
#11179=VERTEX_POINT('',#36471);
#11180=VERTEX_POINT('',#36474);
#11181=VERTEX_POINT('',#36476);
#11182=VERTEX_POINT('',#36478);
#11183=VERTEX_POINT('',#36480);
#11184=VERTEX_POINT('',#36482);
#11185=VERTEX_POINT('',#36484);
#11186=VERTEX_POINT('',#36486);
#11187=VERTEX_POINT('',#36487);
#11188=VERTEX_POINT('',#36489);
#11189=VERTEX_POINT('',#36491);
#11190=VERTEX_POINT('',#36493);
#11191=VERTEX_POINT('',#36495);
#11192=VERTEX_POINT('',#36497);
#11193=VERTEX_POINT('',#36499);
#11194=VERTEX_POINT('',#36501);
#11195=VERTEX_POINT('',#36503);
#11196=VERTEX_POINT('',#36505);
#11197=VERTEX_POINT('',#36507);
#11198=VERTEX_POINT('',#36509);
#11199=VERTEX_POINT('',#36511);
#11200=VERTEX_POINT('',#36513);
#11201=VERTEX_POINT('',#36515);
#11202=VERTEX_POINT('',#36518);
#11203=VERTEX_POINT('',#36521);
#11204=VERTEX_POINT('',#36525);
#11205=VERTEX_POINT('',#36529);
#11206=VERTEX_POINT('',#36533);
#11207=VERTEX_POINT('',#36537);
#11208=VERTEX_POINT('',#36541);
#11209=VERTEX_POINT('',#36545);
#11210=VERTEX_POINT('',#36549);
#11211=VERTEX_POINT('',#36551);
#11212=VERTEX_POINT('',#36555);
#11213=VERTEX_POINT('',#36556);
#11214=VERTEX_POINT('',#36558);
#11215=VERTEX_POINT('',#36560);
#11216=VERTEX_POINT('',#36562);
#11217=VERTEX_POINT('',#36564);
#11218=VERTEX_POINT('',#36566);
#11219=VERTEX_POINT('',#36568);
#11220=VERTEX_POINT('',#36570);
#11221=VERTEX_POINT('',#36572);
#11222=VERTEX_POINT('',#36574);
#11223=VERTEX_POINT('',#36576);
#11224=VERTEX_POINT('',#36578);
#11225=VERTEX_POINT('',#36580);
#11226=VERTEX_POINT('',#36582);
#11227=VERTEX_POINT('',#36584);
#11228=VERTEX_POINT('',#36586);
#11229=VERTEX_POINT('',#36588);
#11230=VERTEX_POINT('',#36590);
#11231=VERTEX_POINT('',#36592);
#11232=VERTEX_POINT('',#36594);
#11233=VERTEX_POINT('',#36596);
#11234=VERTEX_POINT('',#36598);
#11235=VERTEX_POINT('',#36600);
#11236=VERTEX_POINT('',#36603);
#11237=VERTEX_POINT('',#36605);
#11238=VERTEX_POINT('',#36606);
#11239=VERTEX_POINT('',#36608);
#11240=VERTEX_POINT('',#36610);
#11241=VERTEX_POINT('',#36612);
#11242=VERTEX_POINT('',#36614);
#11243=VERTEX_POINT('',#36616);
#11244=VERTEX_POINT('',#36618);
#11245=VERTEX_POINT('',#36620);
#11246=VERTEX_POINT('',#36622);
#11247=VERTEX_POINT('',#36624);
#11248=VERTEX_POINT('',#36626);
#11249=VERTEX_POINT('',#36628);
#11250=VERTEX_POINT('',#36630);
#11251=VERTEX_POINT('',#36632);
#11252=VERTEX_POINT('',#36634);
#11253=VERTEX_POINT('',#36637);
#11254=VERTEX_POINT('',#36639);
#11255=VERTEX_POINT('',#36644);
#11256=VERTEX_POINT('',#36650);
#11257=VERTEX_POINT('',#36656);
#11258=VERTEX_POINT('',#36662);
#11259=VERTEX_POINT('',#36664);
#11260=VERTEX_POINT('',#36668);
#11261=VERTEX_POINT('',#36672);
#11262=VERTEX_POINT('',#36676);
#11263=VERTEX_POINT('',#36680);
#11264=VERTEX_POINT('',#36681);
#11265=VERTEX_POINT('',#36686);
#11266=VERTEX_POINT('',#36690);
#11267=VERTEX_POINT('',#36694);
#11268=VERTEX_POINT('',#36698);
#11269=VERTEX_POINT('',#36702);
#11270=VERTEX_POINT('',#36706);
#11271=VERTEX_POINT('',#36710);
#11272=VERTEX_POINT('',#36714);
#11273=VERTEX_POINT('',#36715);
#11274=VERTEX_POINT('',#36720);
#11275=VERTEX_POINT('',#36724);
#11276=VERTEX_POINT('',#36728);
#11277=VERTEX_POINT('',#36734);
#11278=VERTEX_POINT('',#36738);
#11279=VERTEX_POINT('',#36742);
#11280=VERTEX_POINT('',#36748);
#11281=VERTEX_POINT('',#36752);
#11282=VERTEX_POINT('',#36783);
#11283=VERTEX_POINT('',#36784);
#11284=VERTEX_POINT('',#36789);
#11285=VERTEX_POINT('',#36790);
#11286=VERTEX_POINT('',#36795);
#11287=VERTEX_POINT('',#36796);
#11288=VERTEX_POINT('',#36801);
#11289=VERTEX_POINT('',#36807);
#11290=VERTEX_POINT('',#36808);
#11291=VERTEX_POINT('',#36813);
#11292=VERTEX_POINT('',#36817);
#11293=VERTEX_POINT('',#36821);
#11294=VERTEX_POINT('',#36827);
#11295=VERTEX_POINT('',#36831);
#11296=VERTEX_POINT('',#36835);
#11297=VERTEX_POINT('',#36841);
#13819=EDGE_CURVE('',#11154,#11154,#10338,.T.);
#13820=EDGE_CURVE('',#11154,#11155,#5403,.T.);
#13821=EDGE_CURVE('',#11155,#11155,#10339,.T.);
#13822=EDGE_CURVE('',#11156,#11157,#5404,.T.);
#13823=EDGE_CURVE('',#11158,#11157,#10340,.T.);
#13824=EDGE_CURVE('',#11158,#11159,#5405,.T.);
#13825=EDGE_CURVE('',#11160,#11159,#10341,.T.);
#13826=EDGE_CURVE('',#11160,#11161,#5406,.T.);
#13827=EDGE_CURVE('',#11161,#11162,#5407,.T.);
#13828=EDGE_CURVE('',#11162,#11163,#5408,.T.);
#13829=EDGE_CURVE('',#11163,#11164,#5409,.T.);
#13830=EDGE_CURVE('',#11164,#11165,#5410,.T.);
#13831=EDGE_CURVE('',#11165,#11166,#5411,.T.);
#13832=EDGE_CURVE('',#11166,#11167,#5412,.T.);
#13833=EDGE_CURVE('',#11167,#11168,#5413,.T.);
#13834=EDGE_CURVE('',#11168,#11169,#5414,.T.);
#13835=EDGE_CURVE('',#11170,#11169,#10342,.T.);
#13836=EDGE_CURVE('',#11170,#11171,#5415,.T.);
#13837=EDGE_CURVE('',#11172,#11171,#10343,.T.);
#13838=EDGE_CURVE('',#11172,#11173,#5416,.T.);
#13839=EDGE_CURVE('',#11174,#11173,#5417,.T.);
#13840=EDGE_CURVE('',#11175,#11174,#5418,.T.);
#13841=EDGE_CURVE('',#11176,#11175,#5419,.T.);
#13842=EDGE_CURVE('',#11176,#11177,#5420,.T.);
#13843=EDGE_CURVE('',#11178,#11177,#5421,.T.);
#13844=EDGE_CURVE('',#11179,#11178,#5422,.T.);
#13845=EDGE_CURVE('',#11156,#11179,#5423,.T.);
#13846=EDGE_CURVE('',#11180,#11180,#10344,.T.);
#13847=EDGE_CURVE('',#11181,#11181,#10345,.T.);
#13848=EDGE_CURVE('',#11182,#11182,#10346,.T.);
#13849=EDGE_CURVE('',#11183,#11183,#10347,.T.);
#13850=EDGE_CURVE('',#11184,#11184,#10348,.T.);
#13851=EDGE_CURVE('',#11185,#11185,#10349,.T.);
#13852=EDGE_CURVE('',#11186,#11187,#5424,.T.);
#13853=EDGE_CURVE('',#11187,#11188,#5425,.T.);
#13854=EDGE_CURVE('',#11188,#11189,#10350,.T.);
#13855=EDGE_CURVE('',#11189,#11190,#5426,.T.);
#13856=EDGE_CURVE('',#11190,#11191,#10351,.T.);
#13857=EDGE_CURVE('',#11191,#11192,#5427,.T.);
#13858=EDGE_CURVE('',#11192,#11193,#5428,.T.);
#13859=EDGE_CURVE('',#11193,#11194,#10352,.T.);
#13860=EDGE_CURVE('',#11194,#11195,#5429,.T.);
#13861=EDGE_CURVE('',#11195,#11196,#5430,.T.);
#13862=EDGE_CURVE('',#11196,#11197,#10353,.T.);
#13863=EDGE_CURVE('',#11197,#11198,#5431,.T.);
#13864=EDGE_CURVE('',#11198,#11199,#10354,.T.);
#13865=EDGE_CURVE('',#11199,#11200,#5432,.T.);
#13866=EDGE_CURVE('',#11200,#11201,#5433,.T.);
#13867=EDGE_CURVE('',#11201,#11186,#10355,.T.);
#13868=EDGE_CURVE('',#11202,#11202,#10356,.T.);
#13869=EDGE_CURVE('',#11203,#11203,#10357,.T.);
#13870=EDGE_CURVE('',#11203,#11154,#5434,.T.);
#13871=EDGE_CURVE('',#11204,#11204,#10358,.T.);
#13872=EDGE_CURVE('',#11204,#11180,#5435,.T.);
#13873=EDGE_CURVE('',#11205,#11205,#10359,.T.);
#13874=EDGE_CURVE('',#11205,#11204,#5436,.T.);
#13875=EDGE_CURVE('',#11206,#11206,#10360,.T.);
#13876=EDGE_CURVE('',#11206,#11202,#5437,.T.);
#13877=EDGE_CURVE('',#11207,#11207,#10361,.T.);
#13878=EDGE_CURVE('',#11207,#11206,#5438,.T.);
#13879=EDGE_CURVE('',#11208,#11208,#10362,.T.);
#13880=EDGE_CURVE('',#11208,#11181,#5439,.T.);
#13881=EDGE_CURVE('',#11209,#11209,#10363,.T.);
#13882=EDGE_CURVE('',#11209,#11208,#5440,.T.);
#13883=EDGE_CURVE('',#11210,#11210,#10364,.T.);
#13884=EDGE_CURVE('',#11210,#11211,#5441,.T.);
#13885=EDGE_CURVE('',#11211,#11211,#10365,.T.);
#13886=EDGE_CURVE('',#11212,#11213,#5442,.T.);
#13887=EDGE_CURVE('',#11214,#11212,#10366,.T.);
#13888=EDGE_CURVE('',#11215,#11214,#5443,.T.);
#13889=EDGE_CURVE('',#11216,#11215,#10367,.T.);
#13890=EDGE_CURVE('',#11217,#11216,#5444,.T.);
#13891=EDGE_CURVE('',#11218,#11217,#5445,.T.);
#13892=EDGE_CURVE('',#11219,#11218,#5446,.T.);
#13893=EDGE_CURVE('',#11220,#11219,#5447,.T.);
#13894=EDGE_CURVE('',#11221,#11220,#5448,.T.);
#13895=EDGE_CURVE('',#11222,#11221,#5449,.T.);
#13896=EDGE_CURVE('',#11223,#11222,#5450,.T.);
#13897=EDGE_CURVE('',#11224,#11223,#5451,.T.);
#13898=EDGE_CURVE('',#11225,#11224,#5452,.T.);
#13899=EDGE_CURVE('',#11226,#11225,#10368,.T.);
#13900=EDGE_CURVE('',#11227,#11226,#5453,.T.);
#13901=EDGE_CURVE('',#11228,#11227,#10369,.T.);
#13902=EDGE_CURVE('',#11229,#11228,#5454,.T.);
#13903=EDGE_CURVE('',#11230,#11229,#5455,.T.);
#13904=EDGE_CURVE('',#11231,#11230,#5456,.T.);
#13905=EDGE_CURVE('',#11232,#11231,#5457,.T.);
#13906=EDGE_CURVE('',#11233,#11232,#5458,.T.);
#13907=EDGE_CURVE('',#11234,#11233,#5459,.T.);
#13908=EDGE_CURVE('',#11235,#11234,#5460,.T.);
#13909=EDGE_CURVE('',#11213,#11235,#5461,.T.);
#13910=EDGE_CURVE('',#11236,#11236,#10370,.T.);
#13911=EDGE_CURVE('',#11237,#11238,#5462,.T.);
#13912=EDGE_CURVE('',#11239,#11237,#10371,.T.);
#13913=EDGE_CURVE('',#11240,#11239,#5463,.T.);
#13914=EDGE_CURVE('',#11241,#11240,#10372,.T.);
#13915=EDGE_CURVE('',#11242,#11241,#5464,.T.);
#13916=EDGE_CURVE('',#11243,#11242,#5465,.T.);
#13917=EDGE_CURVE('',#11244,#11243,#10373,.T.);
#13918=EDGE_CURVE('',#11245,#11244,#5466,.T.);
#13919=EDGE_CURVE('',#11246,#11245,#5467,.T.);
#13920=EDGE_CURVE('',#11247,#11246,#10374,.T.);
#13921=EDGE_CURVE('',#11248,#11247,#5468,.T.);
#13922=EDGE_CURVE('',#11249,#11248,#10375,.T.);
#13923=EDGE_CURVE('',#11250,#11249,#5469,.T.);
#13924=EDGE_CURVE('',#11251,#11250,#5470,.T.);
#13925=EDGE_CURVE('',#11252,#11251,#10376,.T.);
#13926=EDGE_CURVE('',#11238,#11252,#5471,.T.);
#13927=EDGE_CURVE('',#11253,#11253,#10377,.T.);
#13928=EDGE_CURVE('',#11254,#11254,#10378,.T.);
#13929=EDGE_CURVE('',#11210,#11185,#5472,.T.);
#13930=EDGE_CURVE('',#11255,#11255,#10379,.T.);
#13931=EDGE_CURVE('',#11255,#11254,#5473,.T.);
#13932=EDGE_CURVE('',#11255,#11184,#5474,.T.);
#13933=EDGE_CURVE('',#11256,#11256,#10380,.T.);
#13934=EDGE_CURVE('',#11256,#11236,#5475,.T.);
#13935=EDGE_CURVE('',#11256,#11183,#5476,.T.);
#13936=EDGE_CURVE('',#11257,#11257,#10381,.T.);
#13937=EDGE_CURVE('',#11257,#11253,#5477,.T.);
#13938=EDGE_CURVE('',#11257,#11182,#5478,.T.);
#13939=EDGE_CURVE('',#11232,#11258,#5479,.T.);
#13940=EDGE_CURVE('',#11258,#11259,#5480,.T.);
#13941=EDGE_CURVE('',#11233,#11259,#5481,.T.);
#13942=EDGE_CURVE('',#11231,#11260,#5482,.T.);
#13943=EDGE_CURVE('',#11260,#11258,#5483,.T.);
#13944=EDGE_CURVE('',#11230,#11261,#5484,.T.);
#13945=EDGE_CURVE('',#11261,#11260,#5485,.T.);
#13946=EDGE_CURVE('',#11229,#11262,#5486,.T.);
#13947=EDGE_CURVE('',#11262,#11261,#5487,.T.);
#13948=EDGE_CURVE('',#11263,#11264,#5488,.T.);
#13949=EDGE_CURVE('',#11264,#11225,#5489,.T.);
#13950=EDGE_CURVE('',#11224,#11263,#5490,.T.);
#13951=EDGE_CURVE('',#11223,#11265,#5491,.T.);
#13952=EDGE_CURVE('',#11265,#11263,#5492,.T.);
#13953=EDGE_CURVE('',#11222,#11266,#5493,.T.);
#13954=EDGE_CURVE('',#11266,#11265,#5494,.T.);
#13955=EDGE_CURVE('',#11221,#11267,#5495,.T.);
#13956=EDGE_CURVE('',#11267,#11266,#5496,.T.);
#13957=EDGE_CURVE('',#11220,#11268,#5497,.T.);
#13958=EDGE_CURVE('',#11268,#11267,#5498,.T.);
#13959=EDGE_CURVE('',#11269,#11268,#5499,.T.);
#13960=EDGE_CURVE('',#11219,#11269,#5500,.T.);
#13961=EDGE_CURVE('',#11270,#11269,#5501,.T.);
#13962=EDGE_CURVE('',#11218,#11270,#5502,.T.);
#13963=EDGE_CURVE('',#11271,#11270,#5503,.T.);
#13964=EDGE_CURVE('',#11217,#11271,#5504,.T.);
#13965=EDGE_CURVE('',#11272,#11273,#5505,.T.);
#13966=EDGE_CURVE('',#11273,#11212,#5506,.T.);
#13967=EDGE_CURVE('',#11213,#11272,#5507,.T.);
#13968=EDGE_CURVE('',#11274,#11214,#5508,.T.);
#13969=EDGE_CURVE('',#11273,#11274,#10382,.T.);
#13970=EDGE_CURVE('',#11275,#11215,#5509,.T.);
#13971=EDGE_CURVE('',#11274,#11275,#5510,.T.);
#13972=EDGE_CURVE('',#11276,#11216,#5511,.T.);
#13973=EDGE_CURVE('',#11275,#11276,#10383,.T.);
#13974=EDGE_CURVE('',#11276,#11271,#5512,.T.);
#13975=EDGE_CURVE('',#11277,#11226,#5513,.T.);
#13976=EDGE_CURVE('',#11264,#11277,#10384,.T.);
#13977=EDGE_CURVE('',#11278,#11227,#5514,.T.);
#13978=EDGE_CURVE('',#11277,#11278,#5515,.T.);
#13979=EDGE_CURVE('',#11279,#11228,#5516,.T.);
#13980=EDGE_CURVE('',#11278,#11279,#10385,.T.);
#13981=EDGE_CURVE('',#11279,#11262,#5517,.T.);
#13982=EDGE_CURVE('',#11280,#11272,#5518,.T.);
#13983=EDGE_CURVE('',#11235,#11280,#5519,.T.);
#13984=EDGE_CURVE('',#11281,#11280,#5520,.T.);
#13985=EDGE_CURVE('',#11234,#11281,#5521,.T.);
#13986=EDGE_CURVE('',#11259,#11281,#5522,.T.);
#13987=EDGE_CURVE('',#11174,#11265,#5523,.T.);
#13988=EDGE_CURVE('',#11263,#11173,#5524,.T.);
#13989=EDGE_CURVE('',#11175,#11266,#5525,.T.);
#13990=EDGE_CURVE('',#11176,#11267,#5526,.T.);
#13991=EDGE_CURVE('',#11268,#11177,#5527,.T.);
#13992=EDGE_CURVE('',#11178,#11269,#5528,.T.);
#13993=EDGE_CURVE('',#11179,#11270,#5529,.T.);
#13994=EDGE_CURVE('',#11156,#11271,#5530,.T.);
#13995=EDGE_CURVE('',#11157,#11276,#5531,.T.);
#13996=EDGE_CURVE('',#11158,#11275,#5532,.T.);
#13997=EDGE_CURVE('',#11159,#11274,#5533,.T.);
#13998=EDGE_CURVE('',#11160,#11273,#5534,.T.);
#13999=EDGE_CURVE('',#11272,#11161,#5535,.T.);
#14000=EDGE_CURVE('',#11282,#11283,#5536,.T.);
#14001=EDGE_CURVE('',#11283,#11251,#5537,.T.);
#14002=EDGE_CURVE('',#11250,#11282,#5538,.T.);
#14003=EDGE_CURVE('',#11284,#11285,#5539,.T.);
#14004=EDGE_CURVE('',#11285,#11246,#5540,.T.);
#14005=EDGE_CURVE('',#11245,#11284,#5541,.T.);
#14006=EDGE_CURVE('',#11286,#11287,#5542,.T.);
#14007=EDGE_CURVE('',#11287,#11243,#5543,.T.);
#14008=EDGE_CURVE('',#11242,#11286,#5544,.T.);
#14009=EDGE_CURVE('',#11288,#11244,#5545,.T.);
#14010=EDGE_CURVE('',#11287,#11288,#10386,.T.);
#14011=EDGE_CURVE('',#11288,#11284,#5546,.T.);
#14012=EDGE_CURVE('',#11289,#11290,#5547,.T.);
#14013=EDGE_CURVE('',#11290,#11237,#5548,.T.);
#14014=EDGE_CURVE('',#11238,#11289,#5549,.T.);
#14015=EDGE_CURVE('',#11291,#11239,#5550,.T.);
#14016=EDGE_CURVE('',#11290,#11291,#10387,.T.);
#14017=EDGE_CURVE('',#11292,#11240,#5551,.T.);
#14018=EDGE_CURVE('',#11291,#11292,#5552,.T.);
#14019=EDGE_CURVE('',#11293,#11241,#5553,.T.);
#14020=EDGE_CURVE('',#11292,#11293,#10388,.T.);
#14021=EDGE_CURVE('',#11293,#11286,#5554,.T.);
#14022=EDGE_CURVE('',#11294,#11247,#5555,.T.);
#14023=EDGE_CURVE('',#11285,#11294,#10389,.T.);
#14024=EDGE_CURVE('',#11295,#11248,#5556,.T.);
#14025=EDGE_CURVE('',#11294,#11295,#5557,.T.);
#14026=EDGE_CURVE('',#11296,#11249,#5558,.T.);
#14027=EDGE_CURVE('',#11295,#11296,#10390,.T.);
#14028=EDGE_CURVE('',#11296,#11282,#5559,.T.);
#14029=EDGE_CURVE('',#11297,#11252,#5560,.T.);
#14030=EDGE_CURVE('',#11283,#11297,#10391,.T.);
#14031=EDGE_CURVE('',#11297,#11289,#5561,.T.);
#14032=EDGE_CURVE('',#11201,#11288,#5562,.T.);
#14033=EDGE_CURVE('',#11284,#11200,#5563,.T.);
#14034=EDGE_CURVE('',#11186,#11287,#5564,.T.);
#14035=EDGE_CURVE('',#11187,#11286,#5565,.T.);
#14036=EDGE_CURVE('',#11188,#11293,#5566,.T.);
#14037=EDGE_CURVE('',#11189,#11292,#5567,.T.);
#14038=EDGE_CURVE('',#11190,#11291,#5568,.T.);
#14039=EDGE_CURVE('',#11191,#11290,#5569,.T.);
#14040=EDGE_CURVE('',#11289,#11192,#5570,.T.);
#14041=EDGE_CURVE('',#11193,#11297,#5571,.T.);
#14042=EDGE_CURVE('',#11195,#11282,#5572,.T.);
#14043=EDGE_CURVE('',#11194,#11283,#5573,.T.);
#14044=EDGE_CURVE('',#11199,#11285,#5574,.T.);
#14045=EDGE_CURVE('',#11196,#11296,#5575,.T.);
#14046=EDGE_CURVE('',#11198,#11294,#5576,.T.);
#14047=EDGE_CURVE('',#11197,#11295,#5577,.T.);
#14048=EDGE_CURVE('',#11162,#11280,#5578,.T.);
#14049=EDGE_CURVE('',#11164,#11259,#5579,.T.);
#14050=EDGE_CURVE('',#11163,#11281,#5580,.T.);
#14051=EDGE_CURVE('',#11258,#11165,#5581,.T.);
#14052=EDGE_CURVE('',#11168,#11262,#5582,.T.);
#14053=EDGE_CURVE('',#11167,#11261,#5583,.T.);
#14054=EDGE_CURVE('',#11166,#11260,#5584,.T.);
#14055=EDGE_CURVE('',#11169,#11279,#5585,.T.);
#14056=EDGE_CURVE('',#11170,#11278,#5586,.T.);
#14057=EDGE_CURVE('',#11171,#11277,#5587,.T.);
#14058=EDGE_CURVE('',#11172,#11264,#5588,.T.);
#17916=ORIENTED_EDGE('',*,*,#13819,.T.);
#17917=ORIENTED_EDGE('',*,*,#13820,.T.);
#17918=ORIENTED_EDGE('',*,*,#13821,.T.);
#17919=ORIENTED_EDGE('',*,*,#13820,.F.);
#17920=ORIENTED_EDGE('',*,*,#13822,.T.);
#17921=ORIENTED_EDGE('',*,*,#13823,.F.);
#17922=ORIENTED_EDGE('',*,*,#13824,.T.);
#17923=ORIENTED_EDGE('',*,*,#13825,.F.);
#17924=ORIENTED_EDGE('',*,*,#13826,.T.);
#17925=ORIENTED_EDGE('',*,*,#13827,.T.);
#17926=ORIENTED_EDGE('',*,*,#13828,.T.);
#17927=ORIENTED_EDGE('',*,*,#13829,.T.);
#17928=ORIENTED_EDGE('',*,*,#13830,.T.);
#17929=ORIENTED_EDGE('',*,*,#13831,.T.);
#17930=ORIENTED_EDGE('',*,*,#13832,.T.);
#17931=ORIENTED_EDGE('',*,*,#13833,.T.);
#17932=ORIENTED_EDGE('',*,*,#13834,.T.);
#17933=ORIENTED_EDGE('',*,*,#13835,.F.);
#17934=ORIENTED_EDGE('',*,*,#13836,.T.);
#17935=ORIENTED_EDGE('',*,*,#13837,.F.);
#17936=ORIENTED_EDGE('',*,*,#13838,.T.);
#17937=ORIENTED_EDGE('',*,*,#13839,.F.);
#17938=ORIENTED_EDGE('',*,*,#13840,.F.);
#17939=ORIENTED_EDGE('',*,*,#13841,.F.);
#17940=ORIENTED_EDGE('',*,*,#13842,.T.);
#17941=ORIENTED_EDGE('',*,*,#13843,.F.);
#17942=ORIENTED_EDGE('',*,*,#13844,.F.);
#17943=ORIENTED_EDGE('',*,*,#13845,.F.);
#17944=ORIENTED_EDGE('',*,*,#13846,.F.);
#17945=ORIENTED_EDGE('',*,*,#13847,.F.);
#17946=ORIENTED_EDGE('',*,*,#13848,.T.);
#17947=ORIENTED_EDGE('',*,*,#13849,.T.);
#17948=ORIENTED_EDGE('',*,*,#13850,.T.);
#17949=ORIENTED_EDGE('',*,*,#13851,.T.);
#17950=ORIENTED_EDGE('',*,*,#13852,.T.);
#17951=ORIENTED_EDGE('',*,*,#13853,.T.);
#17952=ORIENTED_EDGE('',*,*,#13854,.T.);
#17953=ORIENTED_EDGE('',*,*,#13855,.T.);
#17954=ORIENTED_EDGE('',*,*,#13856,.T.);
#17955=ORIENTED_EDGE('',*,*,#13857,.T.);
#17956=ORIENTED_EDGE('',*,*,#13858,.T.);
#17957=ORIENTED_EDGE('',*,*,#13859,.T.);
#17958=ORIENTED_EDGE('',*,*,#13860,.T.);
#17959=ORIENTED_EDGE('',*,*,#13861,.T.);
#17960=ORIENTED_EDGE('',*,*,#13862,.T.);
#17961=ORIENTED_EDGE('',*,*,#13863,.T.);
#17962=ORIENTED_EDGE('',*,*,#13864,.T.);
#17963=ORIENTED_EDGE('',*,*,#13865,.T.);
#17964=ORIENTED_EDGE('',*,*,#13866,.T.);
#17965=ORIENTED_EDGE('',*,*,#13867,.T.);
#17966=ORIENTED_EDGE('',*,*,#13868,.F.);
#17967=ORIENTED_EDGE('',*,*,#13821,.F.);
#17968=ORIENTED_EDGE('',*,*,#13869,.F.);
#17969=ORIENTED_EDGE('',*,*,#13870,.T.);
#17970=ORIENTED_EDGE('',*,*,#13819,.F.);
#17971=ORIENTED_EDGE('',*,*,#13870,.F.);
#17972=ORIENTED_EDGE('',*,*,#13871,.T.);
#17973=ORIENTED_EDGE('',*,*,#13872,.T.);
#17974=ORIENTED_EDGE('',*,*,#13846,.T.);
#17975=ORIENTED_EDGE('',*,*,#13872,.F.);
#17976=ORIENTED_EDGE('',*,*,#13873,.F.);
#17977=ORIENTED_EDGE('',*,*,#13874,.T.);
#17978=ORIENTED_EDGE('',*,*,#13871,.F.);
#17979=ORIENTED_EDGE('',*,*,#13874,.F.);
#17980=ORIENTED_EDGE('',*,*,#13875,.T.);
#17981=ORIENTED_EDGE('',*,*,#13876,.T.);
#17982=ORIENTED_EDGE('',*,*,#13868,.T.);
#17983=ORIENTED_EDGE('',*,*,#13876,.F.);
#17984=ORIENTED_EDGE('',*,*,#13877,.F.);
#17985=ORIENTED_EDGE('',*,*,#13878,.T.);
#17986=ORIENTED_EDGE('',*,*,#13875,.F.);
#17987=ORIENTED_EDGE('',*,*,#13878,.F.);
#17988=ORIENTED_EDGE('',*,*,#13879,.T.);
#17989=ORIENTED_EDGE('',*,*,#13880,.T.);
#17990=ORIENTED_EDGE('',*,*,#13847,.T.);
#17991=ORIENTED_EDGE('',*,*,#13880,.F.);
#17992=ORIENTED_EDGE('',*,*,#13881,.F.);
#17993=ORIENTED_EDGE('',*,*,#13882,.T.);
#17994=ORIENTED_EDGE('',*,*,#13879,.F.);
#17995=ORIENTED_EDGE('',*,*,#13882,.F.);
#17996=ORIENTED_EDGE('',*,*,#13883,.T.);
#17997=ORIENTED_EDGE('',*,*,#13884,.T.);
#17998=ORIENTED_EDGE('',*,*,#13885,.T.);
#17999=ORIENTED_EDGE('',*,*,#13884,.F.);
#18000=ORIENTED_EDGE('',*,*,#13886,.F.);
#18001=ORIENTED_EDGE('',*,*,#13887,.F.);
#18002=ORIENTED_EDGE('',*,*,#13888,.F.);
#18003=ORIENTED_EDGE('',*,*,#13889,.F.);
#18004=ORIENTED_EDGE('',*,*,#13890,.F.);
#18005=ORIENTED_EDGE('',*,*,#13891,.F.);
#18006=ORIENTED_EDGE('',*,*,#13892,.F.);
#18007=ORIENTED_EDGE('',*,*,#13893,.F.);
#18008=ORIENTED_EDGE('',*,*,#13894,.F.);
#18009=ORIENTED_EDGE('',*,*,#13895,.F.);
#18010=ORIENTED_EDGE('',*,*,#13896,.F.);
#18011=ORIENTED_EDGE('',*,*,#13897,.F.);
#18012=ORIENTED_EDGE('',*,*,#13898,.F.);
#18013=ORIENTED_EDGE('',*,*,#13899,.F.);
#18014=ORIENTED_EDGE('',*,*,#13900,.F.);
#18015=ORIENTED_EDGE('',*,*,#13901,.F.);
#18016=ORIENTED_EDGE('',*,*,#13902,.F.);
#18017=ORIENTED_EDGE('',*,*,#13903,.F.);
#18018=ORIENTED_EDGE('',*,*,#13904,.F.);
#18019=ORIENTED_EDGE('',*,*,#13905,.F.);
#18020=ORIENTED_EDGE('',*,*,#13906,.F.);
#18021=ORIENTED_EDGE('',*,*,#13907,.F.);
#18022=ORIENTED_EDGE('',*,*,#13908,.F.);
#18023=ORIENTED_EDGE('',*,*,#13909,.F.);
#18024=ORIENTED_EDGE('',*,*,#13885,.F.);
#18025=ORIENTED_EDGE('',*,*,#13910,.F.);
#18026=ORIENTED_EDGE('',*,*,#13911,.F.);
#18027=ORIENTED_EDGE('',*,*,#13912,.F.);
#18028=ORIENTED_EDGE('',*,*,#13913,.F.);
#18029=ORIENTED_EDGE('',*,*,#13914,.F.);
#18030=ORIENTED_EDGE('',*,*,#13915,.F.);
#18031=ORIENTED_EDGE('',*,*,#13916,.F.);
#18032=ORIENTED_EDGE('',*,*,#13917,.F.);
#18033=ORIENTED_EDGE('',*,*,#13918,.F.);
#18034=ORIENTED_EDGE('',*,*,#13919,.F.);
#18035=ORIENTED_EDGE('',*,*,#13920,.F.);
#18036=ORIENTED_EDGE('',*,*,#13921,.F.);
#18037=ORIENTED_EDGE('',*,*,#13922,.F.);
#18038=ORIENTED_EDGE('',*,*,#13923,.F.);
#18039=ORIENTED_EDGE('',*,*,#13924,.F.);
#18040=ORIENTED_EDGE('',*,*,#13925,.F.);
#18041=ORIENTED_EDGE('',*,*,#13926,.F.);
#18042=ORIENTED_EDGE('',*,*,#13927,.F.);
#18043=ORIENTED_EDGE('',*,*,#13928,.F.);
#18044=ORIENTED_EDGE('',*,*,#13869,.T.);
#18045=ORIENTED_EDGE('',*,*,#13873,.T.);
#18046=ORIENTED_EDGE('',*,*,#13877,.T.);
#18047=ORIENTED_EDGE('',*,*,#13881,.T.);
#18048=ORIENTED_EDGE('',*,*,#13883,.F.);
#18049=ORIENTED_EDGE('',*,*,#13929,.T.);
#18050=ORIENTED_EDGE('',*,*,#13851,.F.);
#18051=ORIENTED_EDGE('',*,*,#13929,.F.);
#18052=ORIENTED_EDGE('',*,*,#13930,.T.);
#18053=ORIENTED_EDGE('',*,*,#13931,.T.);
#18054=ORIENTED_EDGE('',*,*,#13928,.T.);
#18055=ORIENTED_EDGE('',*,*,#13931,.F.);
#18056=ORIENTED_EDGE('',*,*,#13930,.F.);
#18057=ORIENTED_EDGE('',*,*,#13932,.T.);
#18058=ORIENTED_EDGE('',*,*,#13850,.F.);
#18059=ORIENTED_EDGE('',*,*,#13932,.F.);
#18060=ORIENTED_EDGE('',*,*,#13933,.T.);
#18061=ORIENTED_EDGE('',*,*,#13934,.T.);
#18062=ORIENTED_EDGE('',*,*,#13910,.T.);
#18063=ORIENTED_EDGE('',*,*,#13934,.F.);
#18064=ORIENTED_EDGE('',*,*,#13933,.F.);
#18065=ORIENTED_EDGE('',*,*,#13935,.T.);
#18066=ORIENTED_EDGE('',*,*,#13849,.F.);
#18067=ORIENTED_EDGE('',*,*,#13935,.F.);
#18068=ORIENTED_EDGE('',*,*,#13936,.T.);
#18069=ORIENTED_EDGE('',*,*,#13937,.T.);
#18070=ORIENTED_EDGE('',*,*,#13927,.T.);
#18071=ORIENTED_EDGE('',*,*,#13937,.F.);
#18072=ORIENTED_EDGE('',*,*,#13936,.F.);
#18073=ORIENTED_EDGE('',*,*,#13938,.T.);
#18074=ORIENTED_EDGE('',*,*,#13848,.F.);
#18075=ORIENTED_EDGE('',*,*,#13938,.F.);
#18076=ORIENTED_EDGE('',*,*,#13906,.T.);
#18077=ORIENTED_EDGE('',*,*,#13939,.T.);
#18078=ORIENTED_EDGE('',*,*,#13940,.T.);
#18079=ORIENTED_EDGE('',*,*,#13941,.F.);
#18080=ORIENTED_EDGE('',*,*,#13905,.T.);
#18081=ORIENTED_EDGE('',*,*,#13942,.T.);
#18082=ORIENTED_EDGE('',*,*,#13943,.T.);
#18083=ORIENTED_EDGE('',*,*,#13939,.F.);
#18084=ORIENTED_EDGE('',*,*,#13904,.T.);
#18085=ORIENTED_EDGE('',*,*,#13944,.T.);
#18086=ORIENTED_EDGE('',*,*,#13945,.T.);
#18087=ORIENTED_EDGE('',*,*,#13942,.F.);
#18088=ORIENTED_EDGE('',*,*,#13903,.T.);
#18089=ORIENTED_EDGE('',*,*,#13946,.T.);
#18090=ORIENTED_EDGE('',*,*,#13947,.T.);
#18091=ORIENTED_EDGE('',*,*,#13944,.F.);
#18092=ORIENTED_EDGE('',*,*,#13948,.T.);
#18093=ORIENTED_EDGE('',*,*,#13949,.T.);
#18094=ORIENTED_EDGE('',*,*,#13898,.T.);
#18095=ORIENTED_EDGE('',*,*,#13950,.T.);
#18096=ORIENTED_EDGE('',*,*,#13897,.T.);
#18097=ORIENTED_EDGE('',*,*,#13951,.T.);
#18098=ORIENTED_EDGE('',*,*,#13952,.T.);
#18099=ORIENTED_EDGE('',*,*,#13950,.F.);
#18100=ORIENTED_EDGE('',*,*,#13896,.T.);
#18101=ORIENTED_EDGE('',*,*,#13953,.T.);
#18102=ORIENTED_EDGE('',*,*,#13954,.T.);
#18103=ORIENTED_EDGE('',*,*,#13951,.F.);
#18104=ORIENTED_EDGE('',*,*,#13895,.T.);
#18105=ORIENTED_EDGE('',*,*,#13955,.T.);
#18106=ORIENTED_EDGE('',*,*,#13956,.T.);
#18107=ORIENTED_EDGE('',*,*,#13953,.F.);
#18108=ORIENTED_EDGE('',*,*,#13894,.T.);
#18109=ORIENTED_EDGE('',*,*,#13957,.T.);
#18110=ORIENTED_EDGE('',*,*,#13958,.T.);
#18111=ORIENTED_EDGE('',*,*,#13955,.F.);
#18112=ORIENTED_EDGE('',*,*,#13959,.T.);
#18113=ORIENTED_EDGE('',*,*,#13957,.F.);
#18114=ORIENTED_EDGE('',*,*,#13893,.T.);
#18115=ORIENTED_EDGE('',*,*,#13960,.T.);
#18116=ORIENTED_EDGE('',*,*,#13961,.T.);
#18117=ORIENTED_EDGE('',*,*,#13960,.F.);
#18118=ORIENTED_EDGE('',*,*,#13892,.T.);
#18119=ORIENTED_EDGE('',*,*,#13962,.T.);
#18120=ORIENTED_EDGE('',*,*,#13963,.T.);
#18121=ORIENTED_EDGE('',*,*,#13962,.F.);
#18122=ORIENTED_EDGE('',*,*,#13891,.T.);
#18123=ORIENTED_EDGE('',*,*,#13964,.T.);
#18124=ORIENTED_EDGE('',*,*,#13965,.T.);
#18125=ORIENTED_EDGE('',*,*,#13966,.T.);
#18126=ORIENTED_EDGE('',*,*,#13886,.T.);
#18127=ORIENTED_EDGE('',*,*,#13967,.T.);
#18128=ORIENTED_EDGE('',*,*,#13968,.T.);
#18129=ORIENTED_EDGE('',*,*,#13887,.T.);
#18130=ORIENTED_EDGE('',*,*,#13966,.F.);
#18131=ORIENTED_EDGE('',*,*,#13969,.T.);
#18132=ORIENTED_EDGE('',*,*,#13970,.T.);
#18133=ORIENTED_EDGE('',*,*,#13888,.T.);
#18134=ORIENTED_EDGE('',*,*,#13968,.F.);
#18135=ORIENTED_EDGE('',*,*,#13971,.T.);
#18136=ORIENTED_EDGE('',*,*,#13972,.T.);
#18137=ORIENTED_EDGE('',*,*,#13889,.T.);
#18138=ORIENTED_EDGE('',*,*,#13970,.F.);
#18139=ORIENTED_EDGE('',*,*,#13973,.T.);
#18140=ORIENTED_EDGE('',*,*,#13890,.T.);
#18141=ORIENTED_EDGE('',*,*,#13972,.F.);
#18142=ORIENTED_EDGE('',*,*,#13974,.T.);
#18143=ORIENTED_EDGE('',*,*,#13964,.F.);
#18144=ORIENTED_EDGE('',*,*,#13975,.T.);
#18145=ORIENTED_EDGE('',*,*,#13899,.T.);
#18146=ORIENTED_EDGE('',*,*,#13949,.F.);
#18147=ORIENTED_EDGE('',*,*,#13976,.T.);
#18148=ORIENTED_EDGE('',*,*,#13977,.T.);
#18149=ORIENTED_EDGE('',*,*,#13900,.T.);
#18150=ORIENTED_EDGE('',*,*,#13975,.F.);
#18151=ORIENTED_EDGE('',*,*,#13978,.T.);
#18152=ORIENTED_EDGE('',*,*,#13979,.T.);
#18153=ORIENTED_EDGE('',*,*,#13901,.T.);
#18154=ORIENTED_EDGE('',*,*,#13977,.F.);
#18155=ORIENTED_EDGE('',*,*,#13980,.T.);
#18156=ORIENTED_EDGE('',*,*,#13902,.T.);
#18157=ORIENTED_EDGE('',*,*,#13979,.F.);
#18158=ORIENTED_EDGE('',*,*,#13981,.T.);
#18159=ORIENTED_EDGE('',*,*,#13946,.F.);
#18160=ORIENTED_EDGE('',*,*,#13982,.T.);
#18161=ORIENTED_EDGE('',*,*,#13967,.F.);
#18162=ORIENTED_EDGE('',*,*,#13909,.T.);
#18163=ORIENTED_EDGE('',*,*,#13983,.T.);
#18164=ORIENTED_EDGE('',*,*,#13984,.T.);
#18165=ORIENTED_EDGE('',*,*,#13983,.F.);
#18166=ORIENTED_EDGE('',*,*,#13908,.T.);
#18167=ORIENTED_EDGE('',*,*,#13985,.T.);
#18168=ORIENTED_EDGE('',*,*,#13986,.T.);
#18169=ORIENTED_EDGE('',*,*,#13985,.F.);
#18170=ORIENTED_EDGE('',*,*,#13907,.T.);
#18171=ORIENTED_EDGE('',*,*,#13941,.T.);
#18172=ORIENTED_EDGE('',*,*,#13952,.F.);
#18173=ORIENTED_EDGE('',*,*,#13987,.F.);
#18174=ORIENTED_EDGE('',*,*,#13839,.T.);
#18175=ORIENTED_EDGE('',*,*,#13988,.F.);
#18176=ORIENTED_EDGE('',*,*,#13954,.F.);
#18177=ORIENTED_EDGE('',*,*,#13989,.F.);
#18178=ORIENTED_EDGE('',*,*,#13840,.T.);
#18179=ORIENTED_EDGE('',*,*,#13987,.T.);
#18180=ORIENTED_EDGE('',*,*,#13956,.F.);
#18181=ORIENTED_EDGE('',*,*,#13990,.F.);
#18182=ORIENTED_EDGE('',*,*,#13841,.T.);
#18183=ORIENTED_EDGE('',*,*,#13989,.T.);
#18184=ORIENTED_EDGE('',*,*,#13958,.F.);
#18185=ORIENTED_EDGE('',*,*,#13991,.T.);
#18186=ORIENTED_EDGE('',*,*,#13842,.F.);
#18187=ORIENTED_EDGE('',*,*,#13990,.T.);
#18188=ORIENTED_EDGE('',*,*,#13959,.F.);
#18189=ORIENTED_EDGE('',*,*,#13992,.F.);
#18190=ORIENTED_EDGE('',*,*,#13843,.T.);
#18191=ORIENTED_EDGE('',*,*,#13991,.F.);
#18192=ORIENTED_EDGE('',*,*,#13961,.F.);
#18193=ORIENTED_EDGE('',*,*,#13993,.F.);
#18194=ORIENTED_EDGE('',*,*,#13844,.T.);
#18195=ORIENTED_EDGE('',*,*,#13992,.T.);
#18196=ORIENTED_EDGE('',*,*,#13963,.F.);
#18197=ORIENTED_EDGE('',*,*,#13994,.F.);
#18198=ORIENTED_EDGE('',*,*,#13845,.T.);
#18199=ORIENTED_EDGE('',*,*,#13993,.T.);
#18200=ORIENTED_EDGE('',*,*,#13974,.F.);
#18201=ORIENTED_EDGE('',*,*,#13995,.F.);
#18202=ORIENTED_EDGE('',*,*,#13822,.F.);
#18203=ORIENTED_EDGE('',*,*,#13994,.T.);
#18204=ORIENTED_EDGE('',*,*,#13973,.F.);
#18205=ORIENTED_EDGE('',*,*,#13996,.F.);
#18206=ORIENTED_EDGE('',*,*,#13823,.T.);
#18207=ORIENTED_EDGE('',*,*,#13995,.T.);
#18208=ORIENTED_EDGE('',*,*,#13971,.F.);
#18209=ORIENTED_EDGE('',*,*,#13997,.F.);
#18210=ORIENTED_EDGE('',*,*,#13824,.F.);
#18211=ORIENTED_EDGE('',*,*,#13996,.T.);
#18212=ORIENTED_EDGE('',*,*,#13969,.F.);
#18213=ORIENTED_EDGE('',*,*,#13998,.F.);
#18214=ORIENTED_EDGE('',*,*,#13825,.T.);
#18215=ORIENTED_EDGE('',*,*,#13997,.T.);
#18216=ORIENTED_EDGE('',*,*,#13965,.F.);
#18217=ORIENTED_EDGE('',*,*,#13999,.T.);
#18218=ORIENTED_EDGE('',*,*,#13826,.F.);
#18219=ORIENTED_EDGE('',*,*,#13998,.T.);
#18220=ORIENTED_EDGE('',*,*,#14000,.T.);
#18221=ORIENTED_EDGE('',*,*,#14001,.T.);
#18222=ORIENTED_EDGE('',*,*,#13924,.T.);
#18223=ORIENTED_EDGE('',*,*,#14002,.T.);
#18224=ORIENTED_EDGE('',*,*,#14003,.T.);
#18225=ORIENTED_EDGE('',*,*,#14004,.T.);
#18226=ORIENTED_EDGE('',*,*,#13919,.T.);
#18227=ORIENTED_EDGE('',*,*,#14005,.T.);
#18228=ORIENTED_EDGE('',*,*,#14006,.T.);
#18229=ORIENTED_EDGE('',*,*,#14007,.T.);
#18230=ORIENTED_EDGE('',*,*,#13916,.T.);
#18231=ORIENTED_EDGE('',*,*,#14008,.T.);
#18232=ORIENTED_EDGE('',*,*,#14009,.T.);
#18233=ORIENTED_EDGE('',*,*,#13917,.T.);
#18234=ORIENTED_EDGE('',*,*,#14007,.F.);
#18235=ORIENTED_EDGE('',*,*,#14010,.T.);
#18236=ORIENTED_EDGE('',*,*,#13918,.T.);
#18237=ORIENTED_EDGE('',*,*,#14009,.F.);
#18238=ORIENTED_EDGE('',*,*,#14011,.T.);
#18239=ORIENTED_EDGE('',*,*,#14005,.F.);
#18240=ORIENTED_EDGE('',*,*,#14012,.T.);
#18241=ORIENTED_EDGE('',*,*,#14013,.T.);
#18242=ORIENTED_EDGE('',*,*,#13911,.T.);
#18243=ORIENTED_EDGE('',*,*,#14014,.T.);
#18244=ORIENTED_EDGE('',*,*,#14015,.T.);
#18245=ORIENTED_EDGE('',*,*,#13912,.T.);
#18246=ORIENTED_EDGE('',*,*,#14013,.F.);
#18247=ORIENTED_EDGE('',*,*,#14016,.T.);
#18248=ORIENTED_EDGE('',*,*,#14017,.T.);
#18249=ORIENTED_EDGE('',*,*,#13913,.T.);
#18250=ORIENTED_EDGE('',*,*,#14015,.F.);
#18251=ORIENTED_EDGE('',*,*,#14018,.T.);
#18252=ORIENTED_EDGE('',*,*,#14019,.T.);
#18253=ORIENTED_EDGE('',*,*,#13914,.T.);
#18254=ORIENTED_EDGE('',*,*,#14017,.F.);
#18255=ORIENTED_EDGE('',*,*,#14020,.T.);
#18256=ORIENTED_EDGE('',*,*,#13915,.T.);
#18257=ORIENTED_EDGE('',*,*,#14019,.F.);
#18258=ORIENTED_EDGE('',*,*,#14021,.T.);
#18259=ORIENTED_EDGE('',*,*,#14008,.F.);
#18260=ORIENTED_EDGE('',*,*,#14022,.T.);
#18261=ORIENTED_EDGE('',*,*,#13920,.T.);
#18262=ORIENTED_EDGE('',*,*,#14004,.F.);
#18263=ORIENTED_EDGE('',*,*,#14023,.T.);
#18264=ORIENTED_EDGE('',*,*,#14024,.T.);
#18265=ORIENTED_EDGE('',*,*,#13921,.T.);
#18266=ORIENTED_EDGE('',*,*,#14022,.F.);
#18267=ORIENTED_EDGE('',*,*,#14025,.T.);
#18268=ORIENTED_EDGE('',*,*,#14026,.T.);
#18269=ORIENTED_EDGE('',*,*,#13922,.T.);
#18270=ORIENTED_EDGE('',*,*,#14024,.F.);
#18271=ORIENTED_EDGE('',*,*,#14027,.T.);
#18272=ORIENTED_EDGE('',*,*,#13923,.T.);
#18273=ORIENTED_EDGE('',*,*,#14026,.F.);
#18274=ORIENTED_EDGE('',*,*,#14028,.T.);
#18275=ORIENTED_EDGE('',*,*,#14002,.F.);
#18276=ORIENTED_EDGE('',*,*,#14029,.T.);
#18277=ORIENTED_EDGE('',*,*,#13925,.T.);
#18278=ORIENTED_EDGE('',*,*,#14001,.F.);
#18279=ORIENTED_EDGE('',*,*,#14030,.T.);
#18280=ORIENTED_EDGE('',*,*,#13926,.T.);
#18281=ORIENTED_EDGE('',*,*,#14029,.F.);
#18282=ORIENTED_EDGE('',*,*,#14031,.T.);
#18283=ORIENTED_EDGE('',*,*,#14014,.F.);
#18284=ORIENTED_EDGE('',*,*,#14011,.F.);
#18285=ORIENTED_EDGE('',*,*,#14032,.F.);
#18286=ORIENTED_EDGE('',*,*,#13866,.F.);
#18287=ORIENTED_EDGE('',*,*,#14033,.F.);
#18288=ORIENTED_EDGE('',*,*,#14010,.F.);
#18289=ORIENTED_EDGE('',*,*,#14034,.F.);
#18290=ORIENTED_EDGE('',*,*,#13867,.F.);
#18291=ORIENTED_EDGE('',*,*,#14032,.T.);
#18292=ORIENTED_EDGE('',*,*,#14006,.F.);
#18293=ORIENTED_EDGE('',*,*,#14035,.F.);
#18294=ORIENTED_EDGE('',*,*,#13852,.F.);
#18295=ORIENTED_EDGE('',*,*,#14034,.T.);
#18296=ORIENTED_EDGE('',*,*,#14021,.F.);
#18297=ORIENTED_EDGE('',*,*,#14036,.F.);
#18298=ORIENTED_EDGE('',*,*,#13853,.F.);
#18299=ORIENTED_EDGE('',*,*,#14035,.T.);
#18300=ORIENTED_EDGE('',*,*,#14020,.F.);
#18301=ORIENTED_EDGE('',*,*,#14037,.F.);
#18302=ORIENTED_EDGE('',*,*,#13854,.F.);
#18303=ORIENTED_EDGE('',*,*,#14036,.T.);
#18304=ORIENTED_EDGE('',*,*,#14018,.F.);
#18305=ORIENTED_EDGE('',*,*,#14038,.F.);
#18306=ORIENTED_EDGE('',*,*,#13855,.F.);
#18307=ORIENTED_EDGE('',*,*,#14037,.T.);
#18308=ORIENTED_EDGE('',*,*,#14016,.F.);
#18309=ORIENTED_EDGE('',*,*,#14039,.F.);
#18310=ORIENTED_EDGE('',*,*,#13856,.F.);
#18311=ORIENTED_EDGE('',*,*,#14038,.T.);
#18312=ORIENTED_EDGE('',*,*,#14012,.F.);
#18313=ORIENTED_EDGE('',*,*,#14040,.T.);
#18314=ORIENTED_EDGE('',*,*,#13857,.F.);
#18315=ORIENTED_EDGE('',*,*,#14039,.T.);
#18316=ORIENTED_EDGE('',*,*,#14031,.F.);
#18317=ORIENTED_EDGE('',*,*,#14041,.F.);
#18318=ORIENTED_EDGE('',*,*,#13858,.F.);
#18319=ORIENTED_EDGE('',*,*,#14040,.F.);
#18320=ORIENTED_EDGE('',*,*,#14000,.F.);
#18321=ORIENTED_EDGE('',*,*,#14042,.F.);
#18322=ORIENTED_EDGE('',*,*,#13860,.F.);
#18323=ORIENTED_EDGE('',*,*,#14043,.T.);
#18324=ORIENTED_EDGE('',*,*,#14030,.F.);
#18325=ORIENTED_EDGE('',*,*,#14043,.F.);
#18326=ORIENTED_EDGE('',*,*,#13859,.F.);
#18327=ORIENTED_EDGE('',*,*,#14041,.T.);
#18328=ORIENTED_EDGE('',*,*,#14003,.F.);
#18329=ORIENTED_EDGE('',*,*,#14033,.T.);
#18330=ORIENTED_EDGE('',*,*,#13865,.F.);
#18331=ORIENTED_EDGE('',*,*,#14044,.T.);
#18332=ORIENTED_EDGE('',*,*,#14028,.F.);
#18333=ORIENTED_EDGE('',*,*,#14045,.F.);
#18334=ORIENTED_EDGE('',*,*,#13861,.F.);
#18335=ORIENTED_EDGE('',*,*,#14042,.T.);
#18336=ORIENTED_EDGE('',*,*,#14023,.F.);
#18337=ORIENTED_EDGE('',*,*,#14044,.F.);
#18338=ORIENTED_EDGE('',*,*,#13864,.F.);
#18339=ORIENTED_EDGE('',*,*,#14046,.T.);
#18340=ORIENTED_EDGE('',*,*,#14025,.F.);
#18341=ORIENTED_EDGE('',*,*,#14046,.F.);
#18342=ORIENTED_EDGE('',*,*,#13863,.F.);
#18343=ORIENTED_EDGE('',*,*,#14047,.T.);
#18344=ORIENTED_EDGE('',*,*,#14027,.F.);
#18345=ORIENTED_EDGE('',*,*,#14047,.F.);
#18346=ORIENTED_EDGE('',*,*,#13862,.F.);
#18347=ORIENTED_EDGE('',*,*,#14045,.T.);
#18348=ORIENTED_EDGE('',*,*,#13982,.F.);
#18349=ORIENTED_EDGE('',*,*,#14048,.F.);
#18350=ORIENTED_EDGE('',*,*,#13827,.F.);
#18351=ORIENTED_EDGE('',*,*,#13999,.F.);
#18352=ORIENTED_EDGE('',*,*,#13986,.F.);
#18353=ORIENTED_EDGE('',*,*,#14049,.F.);
#18354=ORIENTED_EDGE('',*,*,#13829,.F.);
#18355=ORIENTED_EDGE('',*,*,#14050,.T.);
#18356=ORIENTED_EDGE('',*,*,#13984,.F.);
#18357=ORIENTED_EDGE('',*,*,#14050,.F.);
#18358=ORIENTED_EDGE('',*,*,#13828,.F.);
#18359=ORIENTED_EDGE('',*,*,#14048,.T.);
#18360=ORIENTED_EDGE('',*,*,#13940,.F.);
#18361=ORIENTED_EDGE('',*,*,#14051,.T.);
#18362=ORIENTED_EDGE('',*,*,#13830,.F.);
#18363=ORIENTED_EDGE('',*,*,#14049,.T.);
#18364=ORIENTED_EDGE('',*,*,#13947,.F.);
#18365=ORIENTED_EDGE('',*,*,#14052,.F.);
#18366=ORIENTED_EDGE('',*,*,#13833,.F.);
#18367=ORIENTED_EDGE('',*,*,#14053,.T.);
#18368=ORIENTED_EDGE('',*,*,#13943,.F.);
#18369=ORIENTED_EDGE('',*,*,#14054,.F.);
#18370=ORIENTED_EDGE('',*,*,#13831,.F.);
#18371=ORIENTED_EDGE('',*,*,#14051,.F.);
#18372=ORIENTED_EDGE('',*,*,#13945,.F.);
#18373=ORIENTED_EDGE('',*,*,#14053,.F.);
#18374=ORIENTED_EDGE('',*,*,#13832,.F.);
#18375=ORIENTED_EDGE('',*,*,#14054,.T.);
#18376=ORIENTED_EDGE('',*,*,#13981,.F.);
#18377=ORIENTED_EDGE('',*,*,#14055,.F.);
#18378=ORIENTED_EDGE('',*,*,#13834,.F.);
#18379=ORIENTED_EDGE('',*,*,#14052,.T.);
#18380=ORIENTED_EDGE('',*,*,#13980,.F.);
#18381=ORIENTED_EDGE('',*,*,#14056,.F.);
#18382=ORIENTED_EDGE('',*,*,#13835,.T.);
#18383=ORIENTED_EDGE('',*,*,#14055,.T.);
#18384=ORIENTED_EDGE('',*,*,#13978,.F.);
#18385=ORIENTED_EDGE('',*,*,#14057,.F.);
#18386=ORIENTED_EDGE('',*,*,#13836,.F.);
#18387=ORIENTED_EDGE('',*,*,#14056,.T.);
#18388=ORIENTED_EDGE('',*,*,#13976,.F.);
#18389=ORIENTED_EDGE('',*,*,#14058,.F.);
#18390=ORIENTED_EDGE('',*,*,#13837,.T.);
#18391=ORIENTED_EDGE('',*,*,#14057,.T.);
#18392=ORIENTED_EDGE('',*,*,#13948,.F.);
#18393=ORIENTED_EDGE('',*,*,#13988,.T.);
#18394=ORIENTED_EDGE('',*,*,#13838,.F.);
#18395=ORIENTED_EDGE('',*,*,#14058,.T.);
#25463=CONICAL_SURFACE('',#27208,1.903,0.785398163397448);
#25464=CONICAL_SURFACE('',#27231,1.903,0.785398163397448);
#25465=CONICAL_SURFACE('',#27235,1.903,0.785398163397448);
#25466=CONICAL_SURFACE('',#27239,1.903,0.785398163397448);
#25467=CONICAL_SURFACE('',#27243,1.9525,0.785398163397456);
#25468=CONICAL_SURFACE('',#27261,1.9525,0.785398163397452);
#25469=CONICAL_SURFACE('',#27264,1.9525,0.785398163397452);
#25470=CONICAL_SURFACE('',#27267,1.9525,0.785398163397456);
#25471=CONICAL_SURFACE('',#27283,3.04,0.785398163397456);
#25472=CONICAL_SURFACE('',#27286,3.04,0.785398163397459);
#25473=CONICAL_SURFACE('',#27289,3.04,0.785398163397448);
#25474=CONICAL_SURFACE('',#27292,3.04,0.785398163397448);
#25475=CONICAL_SURFACE('',#27313,2.625,0.785398163397456);
#25476=CONICAL_SURFACE('',#27317,0.949999999999994,0.785398163397451);
#25477=CONICAL_SURFACE('',#27320,0.949999999999994,0.785398163397459);
#25478=CONICAL_SURFACE('',#27323,0.949999999999996,0.785398163397459);
#25479=CONICAL_SURFACE('',#27326,0.949999999999994,0.785398163397451);
#25480=CONICAL_SURFACE('',#27329,2.625,0.785398163397448);
#25618=ADVANCED_FACE('',(#2425),#25463,.F.);
#25619=ADVANCED_FACE('',(#2426,#983,#984,#985,#986,#987,#988,#989,#990,
#991),#1165,.F.);
#25620=ADVANCED_FACE('',(#2427),#2155,.F.);
#25621=ADVANCED_FACE('',(#2428),#25464,.F.);
#25622=ADVANCED_FACE('',(#2429),#2156,.F.);
#25623=ADVANCED_FACE('',(#2430),#25465,.F.);
#25624=ADVANCED_FACE('',(#2431),#2157,.F.);
#25625=ADVANCED_FACE('',(#2432),#25466,.F.);
#25626=ADVANCED_FACE('',(#2433),#2158,.F.);
#25627=ADVANCED_FACE('',(#2434),#25467,.F.);
#25628=ADVANCED_FACE('',(#2435,#992,#993,#994,#995,#996,#997,#998,#999,
#1000),#1166,.T.);
#25629=ADVANCED_FACE('',(#2436),#2159,.F.);
#25630=ADVANCED_FACE('',(#2437),#25468,.F.);
#25631=ADVANCED_FACE('',(#2438),#2160,.F.);
#25632=ADVANCED_FACE('',(#2439),#25469,.F.);
#25633=ADVANCED_FACE('',(#2440),#2161,.F.);
#25634=ADVANCED_FACE('',(#2441),#25470,.F.);
#25635=ADVANCED_FACE('',(#2442),#2162,.F.);
#25636=ADVANCED_FACE('',(#2443),#1167,.T.);
#25637=ADVANCED_FACE('',(#2444),#1168,.T.);
#25638=ADVANCED_FACE('',(#2445),#1169,.T.);
#25639=ADVANCED_FACE('',(#2446),#1170,.T.);
#25640=ADVANCED_FACE('',(#2447),#1171,.T.);
#25641=ADVANCED_FACE('',(#2448),#1172,.T.);
#25642=ADVANCED_FACE('',(#2449),#1173,.T.);
#25643=ADVANCED_FACE('',(#2450),#1174,.T.);
#25644=ADVANCED_FACE('',(#2451),#1175,.T.);
#25645=ADVANCED_FACE('',(#2452),#1176,.T.);
#25646=ADVANCED_FACE('',(#2453),#1177,.T.);
#25647=ADVANCED_FACE('',(#2454),#1178,.T.);
#25648=ADVANCED_FACE('',(#2455),#1179,.T.);
#25649=ADVANCED_FACE('',(#2456),#25471,.T.);
#25650=ADVANCED_FACE('',(#2457),#1180,.T.);
#25651=ADVANCED_FACE('',(#2458),#25472,.T.);
#25652=ADVANCED_FACE('',(#2459),#1181,.T.);
#25653=ADVANCED_FACE('',(#2460),#25473,.T.);
#25654=ADVANCED_FACE('',(#2461),#1182,.T.);
#25655=ADVANCED_FACE('',(#2462),#25474,.T.);
#25656=ADVANCED_FACE('',(#2463),#1183,.T.);
#25657=ADVANCED_FACE('',(#2464),#1184,.T.);
#25658=ADVANCED_FACE('',(#2465),#1185,.T.);
#25659=ADVANCED_FACE('',(#2466),#1186,.T.);
#25660=ADVANCED_FACE('',(#2467),#1187,.T.);
#25661=ADVANCED_FACE('',(#2468),#1188,.T.);
#25662=ADVANCED_FACE('',(#2469),#1189,.T.);
#25663=ADVANCED_FACE('',(#2470),#1190,.T.);
#25664=ADVANCED_FACE('',(#2471),#1191,.T.);
#25665=ADVANCED_FACE('',(#2472),#1192,.T.);
#25666=ADVANCED_FACE('',(#2473),#1193,.T.);
#25667=ADVANCED_FACE('',(#2474),#1194,.T.);
#25668=ADVANCED_FACE('',(#2475),#2163,.T.);
#25669=ADVANCED_FACE('',(#2476),#1195,.T.);
#25670=ADVANCED_FACE('',(#2477),#2164,.T.);
#25671=ADVANCED_FACE('',(#2478),#1196,.T.);
#25672=ADVANCED_FACE('',(#2479),#1197,.T.);
#25673=ADVANCED_FACE('',(#2480),#1198,.T.);
#25674=ADVANCED_FACE('',(#2481),#1199,.T.);
#25675=ADVANCED_FACE('',(#2482),#25475,.F.);
#25676=ADVANCED_FACE('',(#2483),#1200,.T.);
#25677=ADVANCED_FACE('',(#2484),#1201,.T.);
#25678=ADVANCED_FACE('',(#2485),#25476,.F.);
#25679=ADVANCED_FACE('',(#2486),#1202,.T.);
#25680=ADVANCED_FACE('',(#2487),#25477,.F.);
#25681=ADVANCED_FACE('',(#2488),#1203,.T.);
#25682=ADVANCED_FACE('',(#2489),#25478,.F.);
#25683=ADVANCED_FACE('',(#2490),#1204,.T.);
#25684=ADVANCED_FACE('',(#2491),#25479,.F.);
#25685=ADVANCED_FACE('',(#2492),#1205,.T.);
#25686=ADVANCED_FACE('',(#2493),#25480,.F.);
#25687=ADVANCED_FACE('',(#2494),#1206,.T.);
#25688=ADVANCED_FACE('',(#2495),#1207,.F.);
#25689=ADVANCED_FACE('',(#2496),#2165,.F.);
#25690=ADVANCED_FACE('',(#2497),#1208,.F.);
#25691=ADVANCED_FACE('',(#2498),#1209,.F.);
#25692=ADVANCED_FACE('',(#2499),#2166,.F.);
#25693=ADVANCED_FACE('',(#2500),#1210,.F.);
#25694=ADVANCED_FACE('',(#2501),#2167,.F.);
#25695=ADVANCED_FACE('',(#2502),#1211,.F.);
#25696=ADVANCED_FACE('',(#2503),#1212,.F.);
#25697=ADVANCED_FACE('',(#2504),#1213,.F.);
#25698=ADVANCED_FACE('',(#2505),#2168,.F.);
#25699=ADVANCED_FACE('',(#2506),#1214,.F.);
#25700=ADVANCED_FACE('',(#2507),#1215,.F.);
#25701=ADVANCED_FACE('',(#2508),#2169,.F.);
#25702=ADVANCED_FACE('',(#2509),#1216,.F.);
#25703=ADVANCED_FACE('',(#2510),#2170,.F.);
#25704=ADVANCED_FACE('',(#2511),#1217,.T.);
#25705=ADVANCED_FACE('',(#2512),#1218,.T.);
#25706=ADVANCED_FACE('',(#2513),#1219,.T.);
#25707=ADVANCED_FACE('',(#2514),#1220,.T.);
#25708=ADVANCED_FACE('',(#2515),#1221,.T.);
#25709=ADVANCED_FACE('',(#2516),#1222,.T.);
#25710=ADVANCED_FACE('',(#2517),#1223,.T.);
#25711=ADVANCED_FACE('',(#2518),#1224,.T.);
#25712=ADVANCED_FACE('',(#2519),#2171,.T.);
#25713=ADVANCED_FACE('',(#2520),#1225,.T.);
#25714=ADVANCED_FACE('',(#2521),#2172,.T.);
#25715=ADVANCED_FACE('',(#2522),#1226,.T.);
#26930=CLOSED_SHELL('',(#25618,#25619,#25620,#25621,#25622,#25623,#25624,
#25625,#25626,#25627,#25628,#25629,#25630,#25631,#25632,#25633,#25634,#25635,
#25636,#25637,#25638,#25639,#25640,#25641,#25642,#25643,#25644,#25645,#25646,
#25647,#25648,#25649,#25650,#25651,#25652,#25653,#25654,#25655,#25656,#25657,
#25658,#25659,#25660,#25661,#25662,#25663,#25664,#25665,#25666,#25667,#25668,
#25669,#25670,#25671,#25672,#25673,#25674,#25675,#25676,#25677,#25678,#25679,
#25680,#25681,#25682,#25683,#25684,#25685,#25686,#25687,#25688,#25689,#25690,
#25691,#25692,#25693,#25694,#25695,#25696,#25697,#25698,#25699,#25700,#25701,
#25702,#25703,#25704,#25705,#25706,#25707,#25708,#25709,#25710,#25711,#25712,
#25713,#25714,#25715));
#27207=AXIS2_PLACEMENT_3D('',#36418,#29599,#29600);
#27208=AXIS2_PLACEMENT_3D('',#36419,#29601,#29602);
#27209=AXIS2_PLACEMENT_3D('',#36421,#29603,#29604);
#27210=AXIS2_PLACEMENT_3D('',#36424,#29606,#29607);
#27211=AXIS2_PLACEMENT_3D('',#36425,#29608,#29609);
#27212=AXIS2_PLACEMENT_3D('',#36430,#29611,#29612);
#27213=AXIS2_PLACEMENT_3D('',#36434,#29614,#29615);
#27214=AXIS2_PLACEMENT_3D('',#36454,#29625,#29626);
#27215=AXIS2_PLACEMENT_3D('',#36458,#29628,#29629);
#27216=AXIS2_PLACEMENT_3D('',#36475,#29638,#29639);
#27217=AXIS2_PLACEMENT_3D('',#36477,#29640,#29641);
#27218=AXIS2_PLACEMENT_3D('',#36479,#29642,#29643);
#27219=AXIS2_PLACEMENT_3D('',#36481,#29644,#29645);
#27220=AXIS2_PLACEMENT_3D('',#36483,#29646,#29647);
#27221=AXIS2_PLACEMENT_3D('',#36485,#29648,#29649);
#27222=AXIS2_PLACEMENT_3D('',#36492,#29652,#29653);
#27223=AXIS2_PLACEMENT_3D('',#36496,#29655,#29656);
#27224=AXIS2_PLACEMENT_3D('',#36502,#29659,#29660);
#27225=AXIS2_PLACEMENT_3D('',#36508,#29663,#29664);
#27226=AXIS2_PLACEMENT_3D('',#36512,#29666,#29667);
#27227=AXIS2_PLACEMENT_3D('',#36517,#29670,#29671);
#27228=AXIS2_PLACEMENT_3D('',#36519,#29672,#29673);
#27229=AXIS2_PLACEMENT_3D('',#36520,#29674,#29675);
#27230=AXIS2_PLACEMENT_3D('',#36522,#29676,#29677);
#27231=AXIS2_PLACEMENT_3D('',#36524,#29679,#29680);
#27232=AXIS2_PLACEMENT_3D('',#36526,#29681,#29682);
#27233=AXIS2_PLACEMENT_3D('',#36528,#29684,#29685);
#27234=AXIS2_PLACEMENT_3D('',#36530,#29686,#29687);
#27235=AXIS2_PLACEMENT_3D('',#36532,#29689,#29690);
#27236=AXIS2_PLACEMENT_3D('',#36534,#29691,#29692);
#27237=AXIS2_PLACEMENT_3D('',#36536,#29694,#29695);
#27238=AXIS2_PLACEMENT_3D('',#36538,#29696,#29697);
#27239=AXIS2_PLACEMENT_3D('',#36540,#29699,#29700);
#27240=AXIS2_PLACEMENT_3D('',#36542,#29701,#29702);
#27241=AXIS2_PLACEMENT_3D('',#36544,#29704,#29705);
#27242=AXIS2_PLACEMENT_3D('',#36546,#29706,#29707);
#27243=AXIS2_PLACEMENT_3D('',#36548,#29709,#29710);
#27244=AXIS2_PLACEMENT_3D('',#36550,#29711,#29712);
#27245=AXIS2_PLACEMENT_3D('',#36553,#29714,#29715);
#27246=AXIS2_PLACEMENT_3D('',#36554,#29716,#29717);
#27247=AXIS2_PLACEMENT_3D('',#36559,#29719,#29720);
#27248=AXIS2_PLACEMENT_3D('',#36563,#29722,#29723);
#27249=AXIS2_PLACEMENT_3D('',#36583,#29733,#29734);
#27250=AXIS2_PLACEMENT_3D('',#36587,#29736,#29737);
#27251=AXIS2_PLACEMENT_3D('',#36604,#29746,#29747);
#27252=AXIS2_PLACEMENT_3D('',#36609,#29749,#29750);
#27253=AXIS2_PLACEMENT_3D('',#36613,#29752,#29753);
#27254=AXIS2_PLACEMENT_3D('',#36619,#29756,#29757);
#27255=AXIS2_PLACEMENT_3D('',#36625,#29760,#29761);
#27256=AXIS2_PLACEMENT_3D('',#36629,#29763,#29764);
#27257=AXIS2_PLACEMENT_3D('',#36635,#29767,#29768);
#27258=AXIS2_PLACEMENT_3D('',#36638,#29770,#29771);
#27259=AXIS2_PLACEMENT_3D('',#36640,#29772,#29773);
#27260=AXIS2_PLACEMENT_3D('',#36641,#29774,#29775);
#27261=AXIS2_PLACEMENT_3D('',#36643,#29777,#29778);
#27262=AXIS2_PLACEMENT_3D('',#36645,#29779,#29780);
#27263=AXIS2_PLACEMENT_3D('',#36647,#29782,#29783);
#27264=AXIS2_PLACEMENT_3D('',#36649,#29785,#29786);
#27265=AXIS2_PLACEMENT_3D('',#36651,#29787,#29788);
#27266=AXIS2_PLACEMENT_3D('',#36653,#29790,#29791);
#27267=AXIS2_PLACEMENT_3D('',#36655,#29793,#29794);
#27268=AXIS2_PLACEMENT_3D('',#36657,#29795,#29796);
#27269=AXIS2_PLACEMENT_3D('',#36659,#29798,#29799);
#27270=AXIS2_PLACEMENT_3D('',#36661,#29801,#29802);
#27271=AXIS2_PLACEMENT_3D('',#36667,#29806,#29807);
#27272=AXIS2_PLACEMENT_3D('',#36671,#29810,#29811);
#27273=AXIS2_PLACEMENT_3D('',#36675,#29814,#29815);
#27274=AXIS2_PLACEMENT_3D('',#36679,#29818,#29819);
#27275=AXIS2_PLACEMENT_3D('',#36685,#29823,#29824);
#27276=AXIS2_PLACEMENT_3D('',#36689,#29827,#29828);
#27277=AXIS2_PLACEMENT_3D('',#36693,#29831,#29832);
#27278=AXIS2_PLACEMENT_3D('',#36697,#29835,#29836);
#27279=AXIS2_PLACEMENT_3D('',#36701,#29839,#29840);
#27280=AXIS2_PLACEMENT_3D('',#36705,#29843,#29844);
#27281=AXIS2_PLACEMENT_3D('',#36709,#29847,#29848);
#27282=AXIS2_PLACEMENT_3D('',#36713,#29851,#29852);
#27283=AXIS2_PLACEMENT_3D('',#36719,#29856,#29857);
#27284=AXIS2_PLACEMENT_3D('',#36722,#29859,#29860);
#27285=AXIS2_PLACEMENT_3D('',#36723,#29861,#29862);
#27286=AXIS2_PLACEMENT_3D('',#36727,#29865,#29866);
#27287=AXIS2_PLACEMENT_3D('',#36730,#29868,#29869);
#27288=AXIS2_PLACEMENT_3D('',#36731,#29870,#29871);
#27289=AXIS2_PLACEMENT_3D('',#36733,#29873,#29874);
#27290=AXIS2_PLACEMENT_3D('',#36736,#29876,#29877);
#27291=AXIS2_PLACEMENT_3D('',#36737,#29878,#29879);
#27292=AXIS2_PLACEMENT_3D('',#36741,#29882,#29883);
#27293=AXIS2_PLACEMENT_3D('',#36744,#29885,#29886);
#27294=AXIS2_PLACEMENT_3D('',#36745,#29887,#29888);
#27295=AXIS2_PLACEMENT_3D('',#36747,#29890,#29891);
#27296=AXIS2_PLACEMENT_3D('',#36751,#29894,#29895);
#27297=AXIS2_PLACEMENT_3D('',#36755,#29898,#29899);
#27298=AXIS2_PLACEMENT_3D('',#36757,#29901,#29902);
#27299=AXIS2_PLACEMENT_3D('',#36760,#29905,#29906);
#27300=AXIS2_PLACEMENT_3D('',#36762,#29908,#29909);
#27301=AXIS2_PLACEMENT_3D('',#36764,#29911,#29912);
#27302=AXIS2_PLACEMENT_3D('',#36766,#29914,#29915);
#27303=AXIS2_PLACEMENT_3D('',#36768,#29917,#29918);
#27304=AXIS2_PLACEMENT_3D('',#36770,#29920,#29921);
#27305=AXIS2_PLACEMENT_3D('',#36772,#29923,#29924);
#27306=AXIS2_PLACEMENT_3D('',#36774,#29926,#29927);
#27307=AXIS2_PLACEMENT_3D('',#36776,#29929,#29930);
#27308=AXIS2_PLACEMENT_3D('',#36778,#29932,#29933);
#27309=AXIS2_PLACEMENT_3D('',#36780,#29935,#29936);
#27310=AXIS2_PLACEMENT_3D('',#36782,#29938,#29939);
#27311=AXIS2_PLACEMENT_3D('',#36788,#29943,#29944);
#27312=AXIS2_PLACEMENT_3D('',#36794,#29948,#29949);
#27313=AXIS2_PLACEMENT_3D('',#36800,#29953,#29954);
#27314=AXIS2_PLACEMENT_3D('',#36803,#29956,#29957);
#27315=AXIS2_PLACEMENT_3D('',#36804,#29958,#29959);
#27316=AXIS2_PLACEMENT_3D('',#36806,#29961,#29962);
#27317=AXIS2_PLACEMENT_3D('',#36812,#29966,#29967);
#27318=AXIS2_PLACEMENT_3D('',#36815,#29969,#29970);
#27319=AXIS2_PLACEMENT_3D('',#36816,#29971,#29972);
#27320=AXIS2_PLACEMENT_3D('',#36820,#29975,#29976);
#27321=AXIS2_PLACEMENT_3D('',#36823,#29978,#29979);
#27322=AXIS2_PLACEMENT_3D('',#36824,#29980,#29981);
#27323=AXIS2_PLACEMENT_3D('',#36826,#29983,#29984);
#27324=AXIS2_PLACEMENT_3D('',#36829,#29986,#29987);
#27325=AXIS2_PLACEMENT_3D('',#36830,#29988,#29989);
#27326=AXIS2_PLACEMENT_3D('',#36834,#29992,#29993);
#27327=AXIS2_PLACEMENT_3D('',#36837,#29995,#29996);
#27328=AXIS2_PLACEMENT_3D('',#36838,#29997,#29998);
#27329=AXIS2_PLACEMENT_3D('',#36840,#30000,#30001);
#27330=AXIS2_PLACEMENT_3D('',#36843,#30003,#30004);
#27331=AXIS2_PLACEMENT_3D('',#36844,#30005,#30006);
#27332=AXIS2_PLACEMENT_3D('',#36846,#30008,#30009);
#27333=AXIS2_PLACEMENT_3D('',#36849,#30012,#30013);
#27334=AXIS2_PLACEMENT_3D('',#36851,#30015,#30016);
#27335=AXIS2_PLACEMENT_3D('',#36853,#30018,#30019);
#27336=AXIS2_PLACEMENT_3D('',#36855,#30021,#30022);
#27337=AXIS2_PLACEMENT_3D('',#36857,#30024,#30025);
#27338=AXIS2_PLACEMENT_3D('',#36859,#30027,#30028);
#27339=AXIS2_PLACEMENT_3D('',#36861,#30030,#30031);
#27340=AXIS2_PLACEMENT_3D('',#36863,#30033,#30034);
#27341=AXIS2_PLACEMENT_3D('',#36865,#30036,#30037);
#27342=AXIS2_PLACEMENT_3D('',#36868,#30040,#30041);
#27343=AXIS2_PLACEMENT_3D('',#36869,#30042,#30043);
#27344=AXIS2_PLACEMENT_3D('',#36871,#30045,#30046);
#27345=AXIS2_PLACEMENT_3D('',#36873,#30048,#30049);
#27346=AXIS2_PLACEMENT_3D('',#36875,#30051,#30052);
#27347=AXIS2_PLACEMENT_3D('',#36877,#30054,#30055);
#27348=AXIS2_PLACEMENT_3D('',#36878,#30056,#30057);
#27349=AXIS2_PLACEMENT_3D('',#36880,#30059,#30060);
#27350=AXIS2_PLACEMENT_3D('',#36883,#30063,#30064);
#27351=AXIS2_PLACEMENT_3D('',#36884,#30065,#30066);
#27352=AXIS2_PLACEMENT_3D('',#36886,#30068,#30069);
#27353=AXIS2_PLACEMENT_3D('',#36889,#30072,#30073);
#27354=AXIS2_PLACEMENT_3D('',#36891,#30075,#30076);
#27355=AXIS2_PLACEMENT_3D('',#36892,#30077,#30078);
#27356=AXIS2_PLACEMENT_3D('',#36894,#30080,#30081);
#27357=AXIS2_PLACEMENT_3D('',#36896,#30083,#30084);
#27358=AXIS2_PLACEMENT_3D('',#36898,#30086,#30087);
#27359=AXIS2_PLACEMENT_3D('',#36900,#30089,#30090);
#29599=DIRECTION('axis',(0.,0.,1.));
#29600=DIRECTION('refdir',(1.,0.,0.));
#29601=DIRECTION('center_axis',(0.,-1.,0.));
#29602=DIRECTION('ref_axis',(1.,0.,0.));
#29603=DIRECTION('center_axis',(0.,1.,0.));
#29604=DIRECTION('ref_axis',(1.,0.,0.));
#29605=DIRECTION('',(-0.707106781186547,-0.707106781186548,-8.65956056235493E-17));
#29606=DIRECTION('center_axis',(0.,-1.,0.));
#29607=DIRECTION('ref_axis',(1.,0.,0.));
#29608=DIRECTION('center_axis',(0.,1.,0.));
#29609=DIRECTION('ref_axis',(1.,0.,0.));
#29610=DIRECTION('',(1.,0.,0.));
#29611=DIRECTION('center_axis',(0.,1.,0.));
#29612=DIRECTION('ref_axis',(1.,0.,6.96064592241478E-16));
#29613=DIRECTION('',(0.,0.,1.));
#29614=DIRECTION('center_axis',(0.,1.,0.));
#29615=DIRECTION('ref_axis',(2.78425836896591E-15,0.,1.));
#29616=DIRECTION('',(-1.,0.,0.));
#29617=DIRECTION('',(0.,0.,1.));
#29618=DIRECTION('',(-1.,0.,0.));
#29619=DIRECTION('',(0.,0.,-1.));
#29620=DIRECTION('',(-1.,0.,0.));
#29621=DIRECTION('',(0.,0.,1.));
#29622=DIRECTION('',(-1.,0.,0.));
#29623=DIRECTION('',(0.,0.,-1.));
#29624=DIRECTION('',(-1.,0.,0.));
#29625=DIRECTION('center_axis',(0.,1.,0.));
#29626=DIRECTION('ref_axis',(-1.,0.,-2.08819377672444E-15));
#29627=DIRECTION('',(0.,0.,-1.));
#29628=DIRECTION('center_axis',(0.,1.,0.));
#29629=DIRECTION('ref_axis',(-2.78425836896591E-15,0.,-1.));
#29630=DIRECTION('',(1.,0.,0.));
#29631=DIRECTION('',(0.,0.,1.));
#29632=DIRECTION('',(-1.,0.,0.));
#29633=DIRECTION('',(0.,0.,-1.));
#29634=DIRECTION('',(1.,0.,0.));
#29635=DIRECTION('',(0.,0.,1.));
#29636=DIRECTION('',(-1.,0.,0.));
#29637=DIRECTION('',(0.,0.,-1.));
#29638=DIRECTION('center_axis',(0.,-1.,0.));
#29639=DIRECTION('ref_axis',(1.,0.,0.));
#29640=DIRECTION('center_axis',(0.,-1.,0.));
#29641=DIRECTION('ref_axis',(1.,0.,0.));
#29642=DIRECTION('center_axis',(0.,1.,0.));
#29643=DIRECTION('ref_axis',(1.,0.,0.));
#29644=DIRECTION('center_axis',(0.,1.,0.));
#29645=DIRECTION('ref_axis',(1.,0.,0.));
#29646=DIRECTION('center_axis',(0.,1.,0.));
#29647=DIRECTION('ref_axis',(1.,0.,0.));
#29648=DIRECTION('center_axis',(0.,1.,0.));
#29649=DIRECTION('ref_axis',(1.,0.,0.));
#29650=DIRECTION('',(-1.,0.,0.));
#29651=DIRECTION('',(0.,0.,-1.));
#29652=DIRECTION('center_axis',(0.,1.,0.));
#29653=DIRECTION('ref_axis',(1.,0.,8.32667268468876E-15));
#29654=DIRECTION('',(-1.,0.,0.));
#29655=DIRECTION('center_axis',(0.,1.,0.));
#29656=DIRECTION('ref_axis',(8.32667268468874E-15,0.,-1.));
#29657=DIRECTION('',(0.,0.,1.));
#29658=DIRECTION('',(-1.,0.,0.));
#29659=DIRECTION('center_axis',(0.,1.,0.));
#29660=DIRECTION('ref_axis',(8.97149918889015E-16,0.,-1.));
#29661=DIRECTION('',(1.,0.,0.));
#29662=DIRECTION('',(0.,0.,1.));
#29663=DIRECTION('center_axis',(0.,1.,0.));
#29664=DIRECTION('ref_axis',(-1.,0.,-8.32667268468874E-15));
#29665=DIRECTION('',(1.,0.,0.));
#29666=DIRECTION('center_axis',(0.,1.,0.));
#29667=DIRECTION('ref_axis',(-1.11022302462516E-14,0.,1.));
#29668=DIRECTION('',(0.,0.,-1.));
#29669=DIRECTION('',(1.,0.,0.));
#29670=DIRECTION('center_axis',(0.,1.,0.));
#29671=DIRECTION('ref_axis',(-3.58859967555606E-15,0.,1.));
#29672=DIRECTION('center_axis',(0.,-1.,0.));
#29673=DIRECTION('ref_axis',(1.,0.,0.));
#29674=DIRECTION('center_axis',(0.,-1.,0.));
#29675=DIRECTION('ref_axis',(1.,0.,0.));
#29676=DIRECTION('center_axis',(0.,-1.,0.));
#29677=DIRECTION('ref_axis',(1.,0.,0.));
#29678=DIRECTION('',(0.,-1.,0.));
#29679=DIRECTION('center_axis',(0.,-1.,0.));
#29680=DIRECTION('ref_axis',(1.,0.,0.));
#29681=DIRECTION('center_axis',(0.,1.,0.));
#29682=DIRECTION('ref_axis',(1.,0.,0.));
#29683=DIRECTION('',(-0.707106781186547,-0.707106781186548,-8.65956056235493E-17));
#29684=DIRECTION('center_axis',(0.,-1.,0.));
#29685=DIRECTION('ref_axis',(1.,0.,0.));
#29686=DIRECTION('center_axis',(0.,-1.,0.));
#29687=DIRECTION('ref_axis',(1.,0.,0.));
#29688=DIRECTION('',(0.,-1.,0.));
#29689=DIRECTION('center_axis',(0.,-1.,0.));
#29690=DIRECTION('ref_axis',(1.,0.,0.));
#29691=DIRECTION('center_axis',(0.,1.,0.));
#29692=DIRECTION('ref_axis',(1.,0.,0.));
#29693=DIRECTION('',(-0.707106781186547,-0.707106781186548,-8.65956056235493E-17));
#29694=DIRECTION('center_axis',(0.,-1.,0.));
#29695=DIRECTION('ref_axis',(1.,0.,0.));
#29696=DIRECTION('center_axis',(0.,-1.,0.));
#29697=DIRECTION('ref_axis',(1.,0.,0.));
#29698=DIRECTION('',(0.,-1.,0.));
#29699=DIRECTION('center_axis',(0.,-1.,0.));
#29700=DIRECTION('ref_axis',(1.,0.,0.));
#29701=DIRECTION('center_axis',(0.,1.,0.));
#29702=DIRECTION('ref_axis',(1.,0.,0.));
#29703=DIRECTION('',(-0.707106781186547,-0.707106781186548,-8.65956056235493E-17));
#29704=DIRECTION('center_axis',(0.,-1.,0.));
#29705=DIRECTION('ref_axis',(1.,0.,0.));
#29706=DIRECTION('center_axis',(0.,-1.,0.));
#29707=DIRECTION('ref_axis',(1.,0.,0.));
#29708=DIRECTION('',(0.,-1.,0.));
#29709=DIRECTION('center_axis',(0.,1.,0.));
#29710=DIRECTION('ref_axis',(1.,0.,0.));
#29711=DIRECTION('center_axis',(0.,-1.,0.));
#29712=DIRECTION('ref_axis',(1.,0.,0.));
#29713=DIRECTION('',(-0.707106781186553,0.707106781186542,8.659560562355E-17));
#29714=DIRECTION('center_axis',(0.,1.,0.));
#29715=DIRECTION('ref_axis',(1.,0.,0.));
#29716=DIRECTION('center_axis',(0.,1.,0.));
#29717=DIRECTION('ref_axis',(1.,0.,0.));
#29718=DIRECTION('',(-1.,0.,0.));
#29719=DIRECTION('center_axis',(0.,-1.,0.));
#29720=DIRECTION('ref_axis',(2.78425836896591E-15,0.,1.));
#29721=DIRECTION('',(0.,0.,1.));
#29722=DIRECTION('center_axis',(0.,-1.,0.));
#29723=DIRECTION('ref_axis',(1.,0.,6.96064592241478E-16));
#29724=DIRECTION('',(1.,0.,0.));
#29725=DIRECTION('',(0.,0.,1.));
#29726=DIRECTION('',(1.,0.,0.));
#29727=DIRECTION('',(0.,0.,-1.));
#29728=DIRECTION('',(1.,0.,0.));
#29729=DIRECTION('',(0.,0.,1.));
#29730=DIRECTION('',(1.,0.,0.));
#29731=DIRECTION('',(0.,0.,-1.));
#29732=DIRECTION('',(1.,0.,0.));
#29733=DIRECTION('center_axis',(0.,-1.,0.));
#29734=DIRECTION('ref_axis',(-2.78425836896591E-15,0.,-1.));
#29735=DIRECTION('',(0.,0.,-1.));
#29736=DIRECTION('center_axis',(0.,-1.,0.));
#29737=DIRECTION('ref_axis',(-1.,0.,-2.08819377672444E-15));
#29738=DIRECTION('',(-1.,0.,0.));
#29739=DIRECTION('',(0.,0.,-1.));
#29740=DIRECTION('',(-1.,0.,0.));
#29741=DIRECTION('',(0.,0.,1.));
#29742=DIRECTION('',(-1.,0.,0.));
#29743=DIRECTION('',(0.,0.,-1.));
#29744=DIRECTION('',(-1.,0.,0.));
#29745=DIRECTION('',(0.,0.,1.));
#29746=DIRECTION('center_axis',(0.,1.,0.));
#29747=DIRECTION('ref_axis',(1.,0.,0.));
#29748=DIRECTION('',(0.,0.,1.));
#29749=DIRECTION('center_axis',(0.,1.,0.));
#29750=DIRECTION('ref_axis',(8.32667268468873E-15,0.,-1.));
#29751=DIRECTION('',(-1.,0.,0.));
#29752=DIRECTION('center_axis',(0.,1.,0.));
#29753=DIRECTION('ref_axis',(1.,0.,8.32667268468876E-15));
#29754=DIRECTION('',(0.,0.,-1.));
#29755=DIRECTION('',(-1.,0.,0.));
#29756=DIRECTION('center_axis',(0.,1.,0.));
#29757=DIRECTION('ref_axis',(-3.58859967555606E-15,0.,1.));
#29758=DIRECTION('',(1.,0.,0.));
#29759=DIRECTION('',(0.,0.,-1.));
#29760=DIRECTION('center_axis',(0.,1.,0.));
#29761=DIRECTION('ref_axis',(-1.11022302462516E-14,0.,1.));
#29762=DIRECTION('',(1.,0.,0.));
#29763=DIRECTION('center_axis',(0.,1.,0.));
#29764=DIRECTION('ref_axis',(-1.,0.,-8.32667268468873E-15));
#29765=DIRECTION('',(0.,0.,1.));
#29766=DIRECTION('',(1.,0.,0.));
#29767=DIRECTION('center_axis',(0.,1.,0.));
#29768=DIRECTION('ref_axis',(8.97149918889015E-16,0.,-1.));
#29769=DIRECTION('',(-1.,0.,0.));
#29770=DIRECTION('center_axis',(0.,1.,0.));
#29771=DIRECTION('ref_axis',(1.,0.,0.));
#29772=DIRECTION('center_axis',(0.,1.,0.));
#29773=DIRECTION('ref_axis',(1.,0.,0.));
#29774=DIRECTION('center_axis',(0.,-1.,0.));
#29775=DIRECTION('ref_axis',(1.,0.,0.));
#29776=DIRECTION('',(0.,-1.,0.));
#29777=DIRECTION('center_axis',(0.,1.,0.));
#29778=DIRECTION('ref_axis',(1.,0.,0.));
#29779=DIRECTION('center_axis',(0.,-1.,0.));
#29780=DIRECTION('ref_axis',(1.,0.,0.));
#29781=DIRECTION('',(-0.70710678118655,0.707106781186545,8.65956056235497E-17));
#29782=DIRECTION('center_axis',(0.,-1.,0.));
#29783=DIRECTION('ref_axis',(1.,0.,0.));
#29784=DIRECTION('',(0.,-1.,0.));
#29785=DIRECTION('center_axis',(0.,1.,0.));
#29786=DIRECTION('ref_axis',(1.,0.,0.));
#29787=DIRECTION('center_axis',(0.,-1.,0.));
#29788=DIRECTION('ref_axis',(1.,0.,0.));
#29789=DIRECTION('',(-0.70710678118655,0.707106781186545,8.65956056235497E-17));
#29790=DIRECTION('center_axis',(0.,-1.,0.));
#29791=DIRECTION('ref_axis',(1.,0.,0.));
#29792=DIRECTION('',(0.,-1.,0.));
#29793=DIRECTION('center_axis',(0.,1.,0.));
#29794=DIRECTION('ref_axis',(1.,0.,0.));
#29795=DIRECTION('center_axis',(0.,-1.,0.));
#29796=DIRECTION('ref_axis',(1.,0.,0.));
#29797=DIRECTION('',(-0.707106781186553,0.707106781186542,8.659560562355E-17));
#29798=DIRECTION('center_axis',(0.,-1.,0.));
#29799=DIRECTION('ref_axis',(1.,0.,0.));
#29800=DIRECTION('',(0.,-1.,0.));
#29801=DIRECTION('center_axis',(0.,0.70710678118655,0.707106781186545));
#29802=DIRECTION('ref_axis',(1.,0.,0.));
#29803=DIRECTION('',(0.577350269189627,-0.577350269189623,0.577350269189627));
#29804=DIRECTION('',(1.,0.,0.));
#29805=DIRECTION('',(-0.577350269189627,-0.577350269189623,0.577350269189627));
#29806=DIRECTION('center_axis',(0.707106781186544,0.707106781186551,0.));
#29807=DIRECTION('ref_axis',(0.,0.,-1.));
#29808=DIRECTION('',(0.57735026918963,-0.577350269189624,0.577350269189624));
#29809=DIRECTION('',(0.,0.,-1.));
#29810=DIRECTION('center_axis',(0.,0.707106781186548,0.707106781186548));
#29811=DIRECTION('ref_axis',(1.,0.,0.));
#29812=DIRECTION('',(-0.577350269189629,-0.577350269189624,0.577350269189624));
#29813=DIRECTION('',(1.,0.,0.));
#29814=DIRECTION('center_axis',(-0.707106781186545,0.70710678118655,0.));
#29815=DIRECTION('ref_axis',(0.,0.,1.));
#29816=DIRECTION('',(-0.577350269189624,-0.577350269189624,0.577350269189629));
#29817=DIRECTION('',(0.,0.,1.));
#29818=DIRECTION('center_axis',(0.,0.70710678118655,-0.707106781186545));
#29819=DIRECTION('ref_axis',(-1.,0.,0.));
#29820=DIRECTION('',(-1.,0.,0.));
#29821=DIRECTION('',(0.,0.707106781186545,0.70710678118655));
#29822=DIRECTION('',(-0.577350269189624,-0.577350269189624,-0.577350269189629));
#29823=DIRECTION('center_axis',(-0.707106781186545,0.70710678118655,0.));
#29824=DIRECTION('ref_axis',(0.,0.,1.));
#29825=DIRECTION('',(-0.577350269189629,-0.577350269189624,-0.577350269189624));
#29826=DIRECTION('',(0.,0.,1.));
#29827=DIRECTION('center_axis',(0.,0.707106781186548,-0.707106781186548));
#29828=DIRECTION('ref_axis',(-1.,0.,0.));
#29829=DIRECTION('',(0.57735026918963,-0.577350269189624,-0.577350269189624));
#29830=DIRECTION('',(-1.,0.,0.));
#29831=DIRECTION('center_axis',(0.707106781186544,0.707106781186551,0.));
#29832=DIRECTION('ref_axis',(0.,0.,-1.));
#29833=DIRECTION('',(0.57735026918963,-0.577350269189622,-0.577350269189626));
#29834=DIRECTION('',(0.,0.,-1.));
#29835=DIRECTION('center_axis',(0.,0.70710678118655,-0.707106781186545));
#29836=DIRECTION('ref_axis',(-1.,0.,0.));
#29837=DIRECTION('',(-0.577350269189624,-0.577350269189624,-0.577350269189629));
#29838=DIRECTION('',(-1.,0.,0.));
#29839=DIRECTION('center_axis',(-0.707106781186545,0.70710678118655,0.));
#29840=DIRECTION('ref_axis',(0.,0.,1.));
#29841=DIRECTION('',(0.,0.,1.));
#29842=DIRECTION('',(-0.577350269189629,-0.577350269189624,-0.577350269189624));
#29843=DIRECTION('center_axis',(0.,0.707106781186548,-0.707106781186548));
#29844=DIRECTION('ref_axis',(-1.,0.,0.));
#29845=DIRECTION('',(-1.,0.,0.));
#29846=DIRECTION('',(0.577350269189629,-0.577350269189624,-0.577350269189624));
#29847=DIRECTION('center_axis',(0.707106781186545,0.70710678118655,0.));
#29848=DIRECTION('ref_axis',(0.,0.,-1.));
#29849=DIRECTION('',(0.,0.,-1.));
#29850=DIRECTION('',(0.577350269189624,-0.577350269189624,-0.577350269189629));
#29851=DIRECTION('center_axis',(0.,0.70710678118655,0.707106781186545));
#29852=DIRECTION('ref_axis',(1.,0.,0.));
#29853=DIRECTION('',(1.,0.,0.));
#29854=DIRECTION('',(0.,0.707106781186545,-0.70710678118655));
#29855=DIRECTION('',(0.577350269189627,-0.577350269189623,0.577350269189627));
#29856=DIRECTION('center_axis',(0.,-1.,0.));
#29857=DIRECTION('ref_axis',(2.78425836896591E-15,0.,1.));
#29858=DIRECTION('',(-0.707106781186553,0.707106781186542,0.));
#29859=DIRECTION('center_axis',(0.,1.,0.));
#29860=DIRECTION('ref_axis',(2.78425836896591E-15,0.,1.));
#29861=DIRECTION('center_axis',(0.707106781186542,0.707106781186553,0.));
#29862=DIRECTION('ref_axis',(0.,0.,-1.));
#29863=DIRECTION('',(-0.707106781186553,0.707106781186542,-5.23364152894591E-15));
#29864=DIRECTION('',(0.,0.,-1.));
#29865=DIRECTION('center_axis',(0.,-1.,0.));
#29866=DIRECTION('ref_axis',(1.,0.,6.96064592241478E-16));
#29867=DIRECTION('',(0.,0.70710678118654,0.707106781186555));
#29868=DIRECTION('center_axis',(0.,1.,0.));
#29869=DIRECTION('ref_axis',(1.,0.,6.96064592241478E-16));
#29870=DIRECTION('center_axis',(0.,0.70710678118655,-0.707106781186545));
#29871=DIRECTION('ref_axis',(-1.,0.,0.));
#29872=DIRECTION('',(-1.,0.,0.));
#29873=DIRECTION('center_axis',(0.,-1.,0.));
#29874=DIRECTION('ref_axis',(-2.78425836896591E-15,0.,-1.));
#29875=DIRECTION('',(0.707106781186547,0.707106781186547,0.));
#29876=DIRECTION('center_axis',(0.,1.,0.));
#29877=DIRECTION('ref_axis',(-2.78425836896591E-15,0.,-1.));
#29878=DIRECTION('center_axis',(-0.707106781186548,0.707106781186548,0.));
#29879=DIRECTION('ref_axis',(0.,0.,1.));
#29880=DIRECTION('',(0.707106781186547,0.707106781186547,5.23364152894595E-15));
#29881=DIRECTION('',(0.,0.,1.));
#29882=DIRECTION('center_axis',(0.,-1.,0.));
#29883=DIRECTION('ref_axis',(-1.,0.,-2.08819377672444E-15));
#29884=DIRECTION('',(0.,0.707106781186547,-0.707106781186547));
#29885=DIRECTION('center_axis',(0.,1.,0.));
#29886=DIRECTION('ref_axis',(-1.,0.,-2.08819377672444E-15));
#29887=DIRECTION('center_axis',(0.,0.70710678118655,0.707106781186545));
#29888=DIRECTION('ref_axis',(1.,0.,0.));
#29889=DIRECTION('',(1.,0.,0.));
#29890=DIRECTION('center_axis',(0.707106781186545,0.70710678118655,0.));
#29891=DIRECTION('ref_axis',(0.,0.,-1.));
#29892=DIRECTION('',(0.,0.,-1.));
#29893=DIRECTION('',(0.577350269189629,-0.577350269189624,0.577350269189624));
#29894=DIRECTION('center_axis',(0.,0.707106781186548,0.707106781186548));
#29895=DIRECTION('ref_axis',(1.,0.,0.));
#29896=DIRECTION('',(1.,0.,0.));
#29897=DIRECTION('',(-0.577350269189629,-0.577350269189624,0.577350269189624));
#29898=DIRECTION('center_axis',(-0.707106781186545,0.70710678118655,0.));
#29899=DIRECTION('ref_axis',(0.,0.,1.));
#29900=DIRECTION('',(0.,0.,1.));
#29901=DIRECTION('center_axis',(-1.,0.,0.));
#29902=DIRECTION('ref_axis',(0.,0.,1.));
#29903=DIRECTION('',(0.,1.,0.));
#29904=DIRECTION('',(0.,-1.,0.));
#29905=DIRECTION('center_axis',(0.,0.,-1.));
#29906=DIRECTION('ref_axis',(-1.,0.,0.));
#29907=DIRECTION('',(0.,1.,0.));
#29908=DIRECTION('center_axis',(1.,0.,0.));
#29909=DIRECTION('ref_axis',(0.,0.,-1.));
#29910=DIRECTION('',(0.,1.,0.));
#29911=DIRECTION('center_axis',(0.,0.,-1.));
#29912=DIRECTION('ref_axis',(-1.,0.,0.));
#29913=DIRECTION('',(0.,-1.,0.));
#29914=DIRECTION('center_axis',(-1.,0.,0.));
#29915=DIRECTION('ref_axis',(0.,0.,1.));
#29916=DIRECTION('',(0.,1.,0.));
#29917=DIRECTION('center_axis',(0.,0.,-1.));
#29918=DIRECTION('ref_axis',(-1.,0.,0.));
#29919=DIRECTION('',(0.,1.,0.));
#29920=DIRECTION('center_axis',(1.,0.,0.));
#29921=DIRECTION('ref_axis',(0.,0.,-1.));
#29922=DIRECTION('',(0.,1.,0.));
#29923=DIRECTION('center_axis',(0.,0.,-1.));
#29924=DIRECTION('ref_axis',(-1.,0.,0.));
#29925=DIRECTION('',(0.,1.,0.));
#29926=DIRECTION('center_axis',(0.,1.,0.));
#29927=DIRECTION('ref_axis',(1.,0.,6.96064592241478E-16));
#29928=DIRECTION('',(0.,1.,0.));
#29929=DIRECTION('center_axis',(1.,0.,0.));
#29930=DIRECTION('ref_axis',(0.,0.,-1.));
#29931=DIRECTION('',(0.,1.,0.));
#29932=DIRECTION('center_axis',(0.,1.,0.));
#29933=DIRECTION('ref_axis',(2.78425836896591E-15,0.,1.));
#29934=DIRECTION('',(0.,1.,0.));
#29935=DIRECTION('center_axis',(0.,0.,1.));
#29936=DIRECTION('ref_axis',(1.,0.,0.));
#29937=DIRECTION('',(0.,-1.,0.));
#29938=DIRECTION('center_axis',(0.,0.707106781186549,-0.707106781186546));
#29939=DIRECTION('ref_axis',(-1.,0.,0.));
#29940=DIRECTION('',(-1.,0.,0.));
#29941=DIRECTION('',(0.,0.707106781186546,0.707106781186549));
#29942=DIRECTION('',(0.577350269189628,-0.577350269189624,-0.577350269189626));
#29943=DIRECTION('center_axis',(-0.707106781186542,0.707106781186553,0.));
#29944=DIRECTION('ref_axis',(0.,0.,1.));
#29945=DIRECTION('',(0.,0.,1.));
#29946=DIRECTION('',(0.707106781186553,0.707106781186542,0.));
#29947=DIRECTION('',(-0.577350269189631,-0.577350269189622,-0.577350269189624));
#29948=DIRECTION('center_axis',(0.,0.707106781186549,0.707106781186546));
#29949=DIRECTION('ref_axis',(1.,0.,0.));
#29950=DIRECTION('',(1.,0.,0.));
#29951=DIRECTION('',(0.,0.707106781186546,-0.707106781186549));
#29952=DIRECTION('',(-0.577350269189631,-0.577350269189622,0.577350269189624));
#29953=DIRECTION('center_axis',(0.,1.,0.));
#29954=DIRECTION('ref_axis',(-3.58859967555606E-15,0.,1.));
#29955=DIRECTION('',(0.,0.707106781186542,0.707106781186553));
#29956=DIRECTION('center_axis',(0.,-1.,0.));
#29957=DIRECTION('ref_axis',(-3.58859967555606E-15,0.,1.));
#29958=DIRECTION('center_axis',(0.,0.707106781186549,-0.707106781186546));
#29959=DIRECTION('ref_axis',(-1.,0.,0.));
#29960=DIRECTION('',(-1.,0.,0.));
#29961=DIRECTION('center_axis',(0.707106781186545,0.70710678118655,0.));
#29962=DIRECTION('ref_axis',(0.,0.,-1.));
#29963=DIRECTION('',(0.,0.,-1.));
#29964=DIRECTION('',(-0.70710678118655,0.707106781186545,0.));
#29965=DIRECTION('',(0.577350269189628,-0.577350269189624,0.577350269189626));
#29966=DIRECTION('center_axis',(0.,1.,0.));
#29967=DIRECTION('ref_axis',(8.32667268468874E-15,0.,-1.));
#29968=DIRECTION('',(5.23364152894593E-15,0.707106781186545,-0.70710678118655));
#29969=DIRECTION('center_axis',(0.,-1.,0.));
#29970=DIRECTION('ref_axis',(8.32667268468874E-15,0.,-1.));
#29971=DIRECTION('center_axis',(0.,0.70710678118655,0.707106781186545));
#29972=DIRECTION('ref_axis',(1.,0.,0.));
#29973=DIRECTION('',(0.,0.707106781186542,-0.707106781186553));
#29974=DIRECTION('',(1.,0.,0.));
#29975=DIRECTION('center_axis',(0.,1.,0.));
#29976=DIRECTION('ref_axis',(1.,0.,8.32667268468876E-15));
#29977=DIRECTION('',(0.707106781186553,0.707106781186542,5.23364152894591E-15));
#29978=DIRECTION('center_axis',(0.,-1.,0.));
#29979=DIRECTION('ref_axis',(1.,0.,8.32667268468876E-15));
#29980=DIRECTION('center_axis',(-0.707106781186542,0.707106781186553,0.));
#29981=DIRECTION('ref_axis',(0.,0.,1.));
#29982=DIRECTION('',(0.,0.,1.));
#29983=DIRECTION('center_axis',(0.,1.,0.));
#29984=DIRECTION('ref_axis',(-1.11022302462516E-14,0.,1.));
#29985=DIRECTION('',(0.,0.70710678118654,0.707106781186555));
#29986=DIRECTION('center_axis',(0.,-1.,0.));
#29987=DIRECTION('ref_axis',(-1.11022302462516E-14,0.,1.));
#29988=DIRECTION('center_axis',(0.,0.70710678118655,-0.707106781186545));
#29989=DIRECTION('ref_axis',(-1.,0.,0.));
#29990=DIRECTION('',(0.,0.707106781186545,0.70710678118655));
#29991=DIRECTION('',(-1.,0.,0.));
#29992=DIRECTION('center_axis',(0.,1.,0.));
#29993=DIRECTION('ref_axis',(-1.,0.,-8.32667268468874E-15));
#29994=DIRECTION('',(-0.70710678118655,0.707106781186545,-5.23364152894593E-15));
#29995=DIRECTION('center_axis',(0.,-1.,0.));
#29996=DIRECTION('ref_axis',(-1.,0.,-8.32667268468874E-15));
#29997=DIRECTION('center_axis',(0.707106781186545,0.70710678118655,0.));
#29998=DIRECTION('ref_axis',(0.,0.,-1.));
#29999=DIRECTION('',(0.,0.,-1.));
#30000=DIRECTION('center_axis',(0.,1.,0.));
#30001=DIRECTION('ref_axis',(8.97149918889015E-16,0.,-1.));
#30002=DIRECTION('',(0.,0.707106781186547,-0.707106781186547));
#30003=DIRECTION('center_axis',(0.,-1.,0.));
#30004=DIRECTION('ref_axis',(8.97149918889015E-16,0.,-1.));
#30005=DIRECTION('center_axis',(0.,0.707106781186549,0.707106781186546));
#30006=DIRECTION('ref_axis',(1.,0.,0.));
#30007=DIRECTION('',(1.,0.,0.));
#30008=DIRECTION('center_axis',(0.,0.,1.));
#30009=DIRECTION('ref_axis',(1.,0.,0.));
#30010=DIRECTION('',(0.,1.,0.));
#30011=DIRECTION('',(0.,-1.,0.));
#30012=DIRECTION('center_axis',(0.,1.,0.));
#30013=DIRECTION('ref_axis',(-3.58859967555606E-15,0.,1.));
#30014=DIRECTION('',(0.,1.,0.));
#30015=DIRECTION('center_axis',(0.,0.,-1.));
#30016=DIRECTION('ref_axis',(-1.,0.,0.));
#30017=DIRECTION('',(0.,1.,0.));
#30018=DIRECTION('center_axis',(1.,0.,0.));
#30019=DIRECTION('ref_axis',(0.,0.,-1.));
#30020=DIRECTION('',(0.,1.,0.));
#30021=DIRECTION('center_axis',(0.,1.,0.));
#30022=DIRECTION('ref_axis',(1.,0.,8.32667268468876E-15));
#30023=DIRECTION('',(0.,1.,0.));
#30024=DIRECTION('center_axis',(0.,0.,-1.));
#30025=DIRECTION('ref_axis',(-1.,0.,0.));
#30026=DIRECTION('',(0.,1.,0.));
#30027=DIRECTION('center_axis',(0.,1.,0.));
#30028=DIRECTION('ref_axis',(8.32667268468874E-15,0.,-1.));
#30029=DIRECTION('',(0.,1.,0.));
#30030=DIRECTION('center_axis',(-1.,0.,0.));
#30031=DIRECTION('ref_axis',(0.,0.,1.));
#30032=DIRECTION('',(0.,-1.,0.));
#30033=DIRECTION('center_axis',(0.,0.,-1.));
#30034=DIRECTION('ref_axis',(-1.,0.,0.));
#30035=DIRECTION('',(0.,1.,0.));
#30036=DIRECTION('center_axis',(0.,0.,1.));
#30037=DIRECTION('ref_axis',(1.,0.,0.));
#30038=DIRECTION('',(0.,1.,0.));
#30039=DIRECTION('',(0.,1.,0.));
#30040=DIRECTION('center_axis',(0.,1.,0.));
#30041=DIRECTION('ref_axis',(8.97149918889015E-16,0.,-1.));
#30042=DIRECTION('center_axis',(1.,0.,0.));
#30043=DIRECTION('ref_axis',(0.,0.,-1.));
#30044=DIRECTION('',(0.,1.,0.));
#30045=DIRECTION('center_axis',(-1.,0.,0.));
#30046=DIRECTION('ref_axis',(0.,0.,1.));
#30047=DIRECTION('',(0.,1.,0.));
#30048=DIRECTION('center_axis',(0.,1.,0.));
#30049=DIRECTION('ref_axis',(-1.11022302462516E-14,0.,1.));
#30050=DIRECTION('',(0.,1.,0.));
#30051=DIRECTION('center_axis',(0.,0.,1.));
#30052=DIRECTION('ref_axis',(1.,0.,0.));
#30053=DIRECTION('',(0.,1.,0.));
#30054=DIRECTION('center_axis',(0.,1.,0.));
#30055=DIRECTION('ref_axis',(-1.,0.,-8.32667268468874E-15));
#30056=DIRECTION('center_axis',(1.,0.,0.));
#30057=DIRECTION('ref_axis',(0.,0.,-1.));
#30058=DIRECTION('',(0.,1.,0.));
#30059=DIRECTION('center_axis',(-1.,0.,0.));
#30060=DIRECTION('ref_axis',(0.,0.,1.));
#30061=DIRECTION('',(0.,1.,0.));
#30062=DIRECTION('',(0.,1.,0.));
#30063=DIRECTION('center_axis',(0.,0.,1.));
#30064=DIRECTION('ref_axis',(1.,0.,0.));
#30065=DIRECTION('center_axis',(0.,0.,1.));
#30066=DIRECTION('ref_axis',(1.,0.,0.));
#30067=DIRECTION('',(0.,-1.,0.));
#30068=DIRECTION('center_axis',(-1.,0.,0.));
#30069=DIRECTION('ref_axis',(0.,0.,1.));
#30070=DIRECTION('',(0.,1.,0.));
#30071=DIRECTION('',(0.,1.,0.));
#30072=DIRECTION('center_axis',(1.,0.,0.));
#30073=DIRECTION('ref_axis',(0.,0.,-1.));
#30074=DIRECTION('',(0.,1.,0.));
#30075=DIRECTION('center_axis',(0.,0.,1.));
#30076=DIRECTION('ref_axis',(1.,0.,0.));
#30077=DIRECTION('center_axis',(0.,0.,1.));
#30078=DIRECTION('ref_axis',(1.,0.,0.));
#30079=DIRECTION('',(0.,1.,0.));
#30080=DIRECTION('center_axis',(0.,1.,0.));
#30081=DIRECTION('ref_axis',(-1.,0.,-2.08819377672444E-15));
#30082=DIRECTION('',(0.,1.,0.));
#30083=DIRECTION('center_axis',(-1.,0.,0.));
#30084=DIRECTION('ref_axis',(0.,0.,1.));
#30085=DIRECTION('',(0.,1.,0.));
#30086=DIRECTION('center_axis',(0.,1.,0.));
#30087=DIRECTION('ref_axis',(-2.78425836896591E-15,0.,-1.));
#30088=DIRECTION('',(0.,1.,0.));
#30089=DIRECTION('center_axis',(0.,0.,-1.));
#30090=DIRECTION('ref_axis',(-1.,0.,0.));
#36418=CARTESIAN_POINT('',(0.,0.,0.));
#36419=CARTESIAN_POINT('Origin',(13.47,36.061,18.29));
#36420=CARTESIAN_POINT('',(11.692,36.186,18.29));
#36421=CARTESIAN_POINT('Origin',(13.47,36.186,18.29));
#36422=CARTESIAN_POINT('',(11.442,35.936,18.29));
#36423=CARTESIAN_POINT('',(11.567,36.061,18.29));
#36424=CARTESIAN_POINT('Origin',(13.47,35.936,18.29));
#36425=CARTESIAN_POINT('Origin',(15.68,35.936,0.));
#36426=CARTESIAN_POINT('',(17.28,35.936,-17.65));
#36427=CARTESIAN_POINT('',(52.11,35.936,-17.65));
#36428=CARTESIAN_POINT('',(-20.75,35.936,-17.65));
#36429=CARTESIAN_POINT('',(55.3,35.936,-14.46));
#36430=CARTESIAN_POINT('Origin',(52.11,35.936,-14.46));
#36431=CARTESIAN_POINT('',(55.3,35.936,14.46));
#36432=CARTESIAN_POINT('',(55.3,35.936,-14.46));
#36433=CARTESIAN_POINT('',(52.11,35.936,17.65));
#36434=CARTESIAN_POINT('Origin',(52.11,35.936,14.46));
#36435=CARTESIAN_POINT('',(17.28,35.936,17.65));
#36436=CARTESIAN_POINT('',(52.11,35.936,17.65));
#36437=CARTESIAN_POINT('',(17.28,35.936,21.46));
#36438=CARTESIAN_POINT('',(17.28,35.936,17.));
#36439=CARTESIAN_POINT('',(9.66,35.936,21.46));
#36440=CARTESIAN_POINT('',(17.28,35.936,21.46));
#36441=CARTESIAN_POINT('',(9.66,35.936,17.65));
#36442=CARTESIAN_POINT('',(9.66,35.936,21.46));
#36443=CARTESIAN_POINT('',(-9.66,35.936,17.65));
#36444=CARTESIAN_POINT('',(52.11,35.936,17.65));
#36445=CARTESIAN_POINT('',(-9.66,35.936,21.46));
#36446=CARTESIAN_POINT('',(-9.66,35.936,17.));
#36447=CARTESIAN_POINT('',(-17.28,35.936,21.46));
#36448=CARTESIAN_POINT('',(-9.66,35.936,21.46));
#36449=CARTESIAN_POINT('',(-17.28,35.936,17.65));
#36450=CARTESIAN_POINT('',(-17.28,35.936,21.46));
#36451=CARTESIAN_POINT('',(-20.75,35.936,17.65));
#36452=CARTESIAN_POINT('',(52.11,35.936,17.65));
#36453=CARTESIAN_POINT('',(-23.94,35.936,14.46));
#36454=CARTESIAN_POINT('Origin',(-20.75,35.936,14.46));
#36455=CARTESIAN_POINT('',(-23.94,35.936,-14.46));
#36456=CARTESIAN_POINT('',(-23.94,35.936,14.46));
#36457=CARTESIAN_POINT('',(-20.75,35.936,-17.65));
#36458=CARTESIAN_POINT('Origin',(-20.75,35.936,-14.46));
#36459=CARTESIAN_POINT('',(-17.28,35.936,-17.65));
#36460=CARTESIAN_POINT('',(-20.75,35.936,-17.65));
#36461=CARTESIAN_POINT('',(-17.28,35.936,-21.46));
#36462=CARTESIAN_POINT('',(-17.28,35.936,-21.46));
#36463=CARTESIAN_POINT('',(-9.66,35.936,-21.46));
#36464=CARTESIAN_POINT('',(-9.66,35.936,-21.46));
#36465=CARTESIAN_POINT('',(-9.66,35.936,-17.65));
#36466=CARTESIAN_POINT('',(-9.66,35.936,-17.));
#36467=CARTESIAN_POINT('',(9.66,35.936,-17.65));
#36468=CARTESIAN_POINT('',(-20.75,35.936,-17.65));
#36469=CARTESIAN_POINT('',(9.66,35.936,-21.46));
#36470=CARTESIAN_POINT('',(9.66,35.936,-21.46));
#36471=CARTESIAN_POINT('',(17.28,35.936,-21.46));
#36472=CARTESIAN_POINT('',(17.28,35.936,-21.46));
#36473=CARTESIAN_POINT('',(17.28,35.936,-17.));
#36474=CARTESIAN_POINT('',(-15.498,35.936,-18.29));
#36475=CARTESIAN_POINT('Origin',(-13.47,35.936,-18.29));
#36476=CARTESIAN_POINT('',(11.442,35.936,-18.29));
#36477=CARTESIAN_POINT('Origin',(13.47,35.936,-18.29));
#36478=CARTESIAN_POINT('',(47.5375,35.936,-7.87));
#36479=CARTESIAN_POINT('Origin',(49.34,35.936,-7.87));
#36480=CARTESIAN_POINT('',(-19.7825,35.936,7.87));
#36481=CARTESIAN_POINT('Origin',(-17.98,35.936,7.87));
#36482=CARTESIAN_POINT('',(-19.7825,35.936,-7.87));
#36483=CARTESIAN_POINT('Origin',(-17.98,35.936,-7.87));
#36484=CARTESIAN_POINT('',(47.5375,35.936,7.87));
#36485=CARTESIAN_POINT('Origin',(49.34,35.936,7.87));
#36486=CARTESIAN_POINT('',(49.65,35.936,-2.475));
#36487=CARTESIAN_POINT('',(45.52,35.936,-2.475));
#36488=CARTESIAN_POINT('',(32.665,35.936,-2.475));
#36489=CARTESIAN_POINT('',(45.52,35.936,-13.68));
#36490=CARTESIAN_POINT('',(45.52,35.936,6.84));
#36491=CARTESIAN_POINT('',(44.72,35.936,-14.48));
#36492=CARTESIAN_POINT('Origin',(44.72,35.936,-13.68));
#36493=CARTESIAN_POINT('',(-13.36,35.936,-14.48));
#36494=CARTESIAN_POINT('',(30.2,35.936,-14.48));
#36495=CARTESIAN_POINT('',(-14.16,35.936,-13.68));
#36496=CARTESIAN_POINT('Origin',(-13.36,35.936,-13.68));
#36497=CARTESIAN_POINT('',(-14.16,35.936,-2.475));
#36498=CARTESIAN_POINT('',(-14.16,35.936,-6.84));
#36499=CARTESIAN_POINT('',(-18.29,35.936,-2.475));
#36500=CARTESIAN_POINT('',(0.765,35.936,-2.475));
#36501=CARTESIAN_POINT('',(-18.29,35.936,2.475));
#36502=CARTESIAN_POINT('Origin',(-18.29,35.936,0.));
#36503=CARTESIAN_POINT('',(-14.16,35.936,2.475));
#36504=CARTESIAN_POINT('',(-1.305,35.936,2.475));
#36505=CARTESIAN_POINT('',(-14.16,35.936,13.68));
#36506=CARTESIAN_POINT('',(-14.16,35.936,-6.84));
#36507=CARTESIAN_POINT('',(-13.36,35.936,14.48));
#36508=CARTESIAN_POINT('Origin',(-13.36,35.936,13.68));
#36509=CARTESIAN_POINT('',(44.72,35.936,14.48));
#36510=CARTESIAN_POINT('',(1.16,35.936,14.48));
#36511=CARTESIAN_POINT('',(45.52,35.936,13.68));
#36512=CARTESIAN_POINT('Origin',(44.72,35.936,13.68));
#36513=CARTESIAN_POINT('',(45.52,35.936,2.475));
#36514=CARTESIAN_POINT('',(45.52,35.936,6.84));
#36515=CARTESIAN_POINT('',(49.65,35.936,2.475));
#36516=CARTESIAN_POINT('',(30.595,35.936,2.475));
#36517=CARTESIAN_POINT('Origin',(49.65,35.936,0.));
#36518=CARTESIAN_POINT('',(-15.498,35.936,18.29));
#36519=CARTESIAN_POINT('Origin',(-13.47,35.936,18.29));
#36520=CARTESIAN_POINT('Origin',(13.47,39.116,18.29));
#36521=CARTESIAN_POINT('',(11.692,39.116,18.29));
#36522=CARTESIAN_POINT('Origin',(13.47,39.116,18.29));
#36523=CARTESIAN_POINT('',(11.692,39.116,18.29));
#36524=CARTESIAN_POINT('Origin',(-13.47,36.061,-18.29));
#36525=CARTESIAN_POINT('',(-15.248,36.186,-18.29));
#36526=CARTESIAN_POINT('Origin',(-13.47,36.186,-18.29));
#36527=CARTESIAN_POINT('',(-15.373,36.061,-18.29));
#36528=CARTESIAN_POINT('Origin',(-13.47,39.116,-18.29));
#36529=CARTESIAN_POINT('',(-15.248,39.116,-18.29));
#36530=CARTESIAN_POINT('Origin',(-13.47,39.116,-18.29));
#36531=CARTESIAN_POINT('',(-15.248,39.116,-18.29));
#36532=CARTESIAN_POINT('Origin',(-13.47,36.061,18.29));
#36533=CARTESIAN_POINT('',(-15.248,36.186,18.29));
#36534=CARTESIAN_POINT('Origin',(-13.47,36.186,18.29));
#36535=CARTESIAN_POINT('',(-15.373,36.061,18.29));
#36536=CARTESIAN_POINT('Origin',(-13.47,39.116,18.29));
#36537=CARTESIAN_POINT('',(-15.248,39.116,18.29));
#36538=CARTESIAN_POINT('Origin',(-13.47,39.116,18.29));
#36539=CARTESIAN_POINT('',(-15.248,39.116,18.29));
#36540=CARTESIAN_POINT('Origin',(13.47,36.061,-18.29));
#36541=CARTESIAN_POINT('',(11.692,36.186,-18.29));
#36542=CARTESIAN_POINT('Origin',(13.47,36.186,-18.29));
#36543=CARTESIAN_POINT('',(11.567,36.061,-18.29));
#36544=CARTESIAN_POINT('Origin',(13.47,39.116,-18.29));
#36545=CARTESIAN_POINT('',(11.692,39.116,-18.29));
#36546=CARTESIAN_POINT('Origin',(13.47,39.116,-18.29));
#36547=CARTESIAN_POINT('',(11.692,39.116,-18.29));
#36548=CARTESIAN_POINT('Origin',(49.34,38.966,7.87));
#36549=CARTESIAN_POINT('',(47.5375,38.816,7.87));
#36550=CARTESIAN_POINT('Origin',(49.34,38.816,7.87));
#36551=CARTESIAN_POINT('',(47.2375,39.116,7.87));
#36552=CARTESIAN_POINT('',(47.3875,38.966,7.87));
#36553=CARTESIAN_POINT('Origin',(49.34,39.116,7.87));
#36554=CARTESIAN_POINT('Origin',(15.68,39.116,0.));
#36555=CARTESIAN_POINT('',(52.11,39.116,17.35));
#36556=CARTESIAN_POINT('',(16.98,39.116,17.35));
#36557=CARTESIAN_POINT('',(-2.535,39.116,17.35));
#36558=CARTESIAN_POINT('',(55.,39.116,14.46));
#36559=CARTESIAN_POINT('Origin',(52.11,39.116,14.46));
#36560=CARTESIAN_POINT('',(55.,39.116,-14.46));
#36561=CARTESIAN_POINT('',(55.,39.116,7.23));
#36562=CARTESIAN_POINT('',(52.11,39.116,-17.35));
#36563=CARTESIAN_POINT('Origin',(52.11,39.116,-14.46));
#36564=CARTESIAN_POINT('',(16.98,39.116,-17.35));
#36565=CARTESIAN_POINT('',(33.895,39.116,-17.35));
#36566=CARTESIAN_POINT('',(16.98,39.116,-21.16));
#36567=CARTESIAN_POINT('',(16.98,39.116,-8.5));
#36568=CARTESIAN_POINT('',(9.96,39.116,-21.16));
#36569=CARTESIAN_POINT('',(16.48,39.116,-21.16));
#36570=CARTESIAN_POINT('',(9.96,39.116,-17.35));
#36571=CARTESIAN_POINT('',(9.96,39.116,-10.73));
#36572=CARTESIAN_POINT('',(-9.96,39.116,-17.35));
#36573=CARTESIAN_POINT('',(33.895,39.116,-17.35));
#36574=CARTESIAN_POINT('',(-9.96,39.116,-21.16));
#36575=CARTESIAN_POINT('',(-9.96,39.116,-8.5));
#36576=CARTESIAN_POINT('',(-16.98,39.116,-21.16));
#36577=CARTESIAN_POINT('',(3.01,39.116,-21.16));
#36578=CARTESIAN_POINT('',(-16.98,39.116,-17.35));
#36579=CARTESIAN_POINT('',(-16.98,39.116,-10.73));
#36580=CARTESIAN_POINT('',(-20.75,39.116,-17.35));
#36581=CARTESIAN_POINT('',(33.895,39.116,-17.35));
#36582=CARTESIAN_POINT('',(-23.64,39.116,-14.46));
#36583=CARTESIAN_POINT('Origin',(-20.75,39.116,-14.46));
#36584=CARTESIAN_POINT('',(-23.64,39.116,14.46));
#36585=CARTESIAN_POINT('',(-23.64,39.116,-7.23));
#36586=CARTESIAN_POINT('',(-20.75,39.116,17.35));
#36587=CARTESIAN_POINT('Origin',(-20.75,39.116,14.46));
#36588=CARTESIAN_POINT('',(-16.98,39.116,17.35));
#36589=CARTESIAN_POINT('',(-2.535,39.116,17.35));
#36590=CARTESIAN_POINT('',(-16.98,39.116,21.16));
#36591=CARTESIAN_POINT('',(-16.98,39.116,8.5));
#36592=CARTESIAN_POINT('',(-9.96,39.116,21.16));
#36593=CARTESIAN_POINT('',(-0.800000000000002,39.116,21.16));
#36594=CARTESIAN_POINT('',(-9.96,39.116,17.35));
#36595=CARTESIAN_POINT('',(-9.96,39.116,10.73));
#36596=CARTESIAN_POINT('',(9.96,39.116,17.35));
#36597=CARTESIAN_POINT('',(-2.535,39.116,17.35));
#36598=CARTESIAN_POINT('',(9.96,39.116,21.16));
#36599=CARTESIAN_POINT('',(9.96,39.116,8.5));
#36600=CARTESIAN_POINT('',(16.98,39.116,21.16));
#36601=CARTESIAN_POINT('',(12.67,39.116,21.16));
#36602=CARTESIAN_POINT('',(16.98,39.116,10.73));
#36603=CARTESIAN_POINT('',(-20.0825,39.116,7.87));
#36604=CARTESIAN_POINT('Origin',(-17.98,39.116,7.87));
#36605=CARTESIAN_POINT('',(-14.46,39.116,-13.68));
#36606=CARTESIAN_POINT('',(-14.46,39.116,-2.775));
#36607=CARTESIAN_POINT('',(-14.46,39.116,-6.84));
#36608=CARTESIAN_POINT('',(-13.36,39.116,-14.78));
#36609=CARTESIAN_POINT('Origin',(-13.36,39.116,-13.68));
#36610=CARTESIAN_POINT('',(44.72,39.116,-14.78));
#36611=CARTESIAN_POINT('',(30.2,39.116,-14.78));
#36612=CARTESIAN_POINT('',(45.82,39.116,-13.68));
#36613=CARTESIAN_POINT('Origin',(44.72,39.116,-13.68));
#36614=CARTESIAN_POINT('',(45.82,39.116,-2.775));
#36615=CARTESIAN_POINT('',(45.82,39.116,6.84));
#36616=CARTESIAN_POINT('',(49.65,39.116,-2.775));
#36617=CARTESIAN_POINT('',(32.665,39.116,-2.775));
#36618=CARTESIAN_POINT('',(49.65,39.116,2.775));
#36619=CARTESIAN_POINT('Origin',(49.65,39.116,0.));
#36620=CARTESIAN_POINT('',(45.82,39.116,2.775));
#36621=CARTESIAN_POINT('',(30.595,39.116,2.775));
#36622=CARTESIAN_POINT('',(45.82,39.116,13.68));
#36623=CARTESIAN_POINT('',(45.82,39.116,6.84));
#36624=CARTESIAN_POINT('',(44.72,39.116,14.78));
#36625=CARTESIAN_POINT('Origin',(44.72,39.116,13.68));
#36626=CARTESIAN_POINT('',(-13.36,39.116,14.78));
#36627=CARTESIAN_POINT('',(1.16,39.116,14.78));
#36628=CARTESIAN_POINT('',(-14.46,39.116,13.68));
#36629=CARTESIAN_POINT('Origin',(-13.36,39.116,13.68));
#36630=CARTESIAN_POINT('',(-14.46,39.116,2.775));
#36631=CARTESIAN_POINT('',(-14.46,39.116,-6.84));
#36632=CARTESIAN_POINT('',(-18.29,39.116,2.775));
#36633=CARTESIAN_POINT('',(-1.305,39.116,2.775));
#36634=CARTESIAN_POINT('',(-18.29,39.116,-2.775));
#36635=CARTESIAN_POINT('Origin',(-18.29,39.116,0.));
#36636=CARTESIAN_POINT('',(0.765,39.116,-2.775));
#36637=CARTESIAN_POINT('',(47.2375,39.116,-7.87));
#36638=CARTESIAN_POINT('Origin',(49.34,39.116,-7.87));
#36639=CARTESIAN_POINT('',(-20.0825,39.116,-7.87));
#36640=CARTESIAN_POINT('Origin',(-17.98,39.116,-7.87));
#36641=CARTESIAN_POINT('Origin',(49.34,39.116,7.87));
#36642=CARTESIAN_POINT('',(47.5375,39.116,7.87));
#36643=CARTESIAN_POINT('Origin',(-17.98,38.966,-7.87));
#36644=CARTESIAN_POINT('',(-19.7825,38.816,-7.87));
#36645=CARTESIAN_POINT('Origin',(-17.98,38.816,-7.87));
#36646=CARTESIAN_POINT('',(-19.9325,38.966,-7.87));
#36647=CARTESIAN_POINT('Origin',(-17.98,39.116,-7.87));
#36648=CARTESIAN_POINT('',(-19.7825,39.116,-7.87));
#36649=CARTESIAN_POINT('Origin',(-17.98,38.966,7.87));
#36650=CARTESIAN_POINT('',(-19.7825,38.816,7.87));
#36651=CARTESIAN_POINT('Origin',(-17.98,38.816,7.87));
#36652=CARTESIAN_POINT('',(-19.9325,38.966,7.87));
#36653=CARTESIAN_POINT('Origin',(-17.98,39.116,7.87));
#36654=CARTESIAN_POINT('',(-19.7825,39.116,7.87));
#36655=CARTESIAN_POINT('Origin',(49.34,38.966,-7.87));
#36656=CARTESIAN_POINT('',(47.5375,38.816,-7.87));
#36657=CARTESIAN_POINT('Origin',(49.34,38.816,-7.87));
#36658=CARTESIAN_POINT('',(47.3875,38.966,-7.87));
#36659=CARTESIAN_POINT('Origin',(49.34,39.116,-7.87));
#36660=CARTESIAN_POINT('',(47.5375,39.116,-7.87));
#36661=CARTESIAN_POINT('Origin',(-2.535,38.966,17.5));
#36662=CARTESIAN_POINT('',(-9.66,38.816,17.65));
#36663=CARTESIAN_POINT('',(-9.96,39.116,17.35));
#36664=CARTESIAN_POINT('',(9.66,38.816,17.65));
#36665=CARTESIAN_POINT('',(-2.535,38.816,17.65));
#36666=CARTESIAN_POINT('',(9.96,39.116,17.35));
#36667=CARTESIAN_POINT('Origin',(-9.81,38.966,10.73));
#36668=CARTESIAN_POINT('',(-9.66,38.816,21.46));
#36669=CARTESIAN_POINT('',(-9.96,39.116,21.16));
#36670=CARTESIAN_POINT('',(-9.66,38.816,10.73));
#36671=CARTESIAN_POINT('Origin',(-0.800000000000002,38.966,21.31));
#36672=CARTESIAN_POINT('',(-17.28,38.816,21.46));
#36673=CARTESIAN_POINT('',(-16.98,39.116,21.16));
#36674=CARTESIAN_POINT('',(-0.800000000000002,38.816,21.46));
#36675=CARTESIAN_POINT('Origin',(-17.13,38.966,8.5));
#36676=CARTESIAN_POINT('',(-17.28,38.816,17.65));
#36677=CARTESIAN_POINT('',(-16.98,39.116,17.35));
#36678=CARTESIAN_POINT('',(-17.28,38.816,8.5));
#36679=CARTESIAN_POINT('Origin',(33.895,38.966,-17.5));
#36680=CARTESIAN_POINT('',(-17.28,38.816,-17.65));
#36681=CARTESIAN_POINT('',(-20.75,38.816,-17.65));
#36682=CARTESIAN_POINT('',(33.895,38.816,-17.65));
#36683=CARTESIAN_POINT('',(-20.75,38.816,-17.65));
#36684=CARTESIAN_POINT('',(-16.98,39.116,-17.35));
#36685=CARTESIAN_POINT('Origin',(-17.13,38.966,-10.73));
#36686=CARTESIAN_POINT('',(-17.28,38.816,-21.46));
#36687=CARTESIAN_POINT('',(-16.98,39.116,-21.16));
#36688=CARTESIAN_POINT('',(-17.28,38.816,-10.73));
#36689=CARTESIAN_POINT('Origin',(3.01,38.966,-21.31));
#36690=CARTESIAN_POINT('',(-9.66,38.816,-21.46));
#36691=CARTESIAN_POINT('',(-9.96,39.116,-21.16));
#36692=CARTESIAN_POINT('',(3.01,38.816,-21.46));
#36693=CARTESIAN_POINT('Origin',(-9.81,38.966,-8.5));
#36694=CARTESIAN_POINT('',(-9.66,38.816,-17.65));
#36695=CARTESIAN_POINT('',(-9.96,39.116,-17.35));
#36696=CARTESIAN_POINT('',(-9.66,38.816,-8.5));
#36697=CARTESIAN_POINT('Origin',(33.895,38.966,-17.5));
#36698=CARTESIAN_POINT('',(9.66,38.816,-17.65));
#36699=CARTESIAN_POINT('',(9.96,39.116,-17.35));
#36700=CARTESIAN_POINT('',(33.895,38.816,-17.65));
#36701=CARTESIAN_POINT('Origin',(9.81,38.966,-10.73));
#36702=CARTESIAN_POINT('',(9.66,38.816,-21.46));
#36703=CARTESIAN_POINT('',(9.66,38.816,-10.73));
#36704=CARTESIAN_POINT('',(9.96,39.116,-21.16));
#36705=CARTESIAN_POINT('Origin',(16.48,38.966,-21.31));
#36706=CARTESIAN_POINT('',(17.28,38.816,-21.46));
#36707=CARTESIAN_POINT('',(16.48,38.816,-21.46));
#36708=CARTESIAN_POINT('',(16.98,39.116,-21.16));
#36709=CARTESIAN_POINT('Origin',(17.13,38.966,-8.5));
#36710=CARTESIAN_POINT('',(17.28,38.816,-17.65));
#36711=CARTESIAN_POINT('',(17.28,38.816,-8.5));
#36712=CARTESIAN_POINT('',(16.98,39.116,-17.35));
#36713=CARTESIAN_POINT('Origin',(-2.535,38.966,17.5));
#36714=CARTESIAN_POINT('',(17.28,38.816,17.65));
#36715=CARTESIAN_POINT('',(52.11,38.816,17.65));
#36716=CARTESIAN_POINT('',(-2.535,38.816,17.65));
#36717=CARTESIAN_POINT('',(52.11,38.816,17.65));
#36718=CARTESIAN_POINT('',(16.98,39.116,17.35));
#36719=CARTESIAN_POINT('Origin',(52.11,38.966,14.46));
#36720=CARTESIAN_POINT('',(55.3,38.816,14.46));
#36721=CARTESIAN_POINT('',(55.3,38.816,14.46));
#36722=CARTESIAN_POINT('Origin',(52.11,38.816,14.46));
#36723=CARTESIAN_POINT('Origin',(55.15,38.966,7.23));
#36724=CARTESIAN_POINT('',(55.3,38.816,-14.46));
#36725=CARTESIAN_POINT('',(55.3,38.816,-14.46));
#36726=CARTESIAN_POINT('',(55.3,38.816,7.23));
#36727=CARTESIAN_POINT('Origin',(52.11,38.966,-14.46));
#36728=CARTESIAN_POINT('',(52.11,38.816,-17.65));
#36729=CARTESIAN_POINT('',(52.11,38.816,-17.65));
#36730=CARTESIAN_POINT('Origin',(52.11,38.816,-14.46));
#36731=CARTESIAN_POINT('Origin',(33.895,38.966,-17.5));
#36732=CARTESIAN_POINT('',(33.895,38.816,-17.65));
#36733=CARTESIAN_POINT('Origin',(-20.75,38.966,-14.46));
#36734=CARTESIAN_POINT('',(-23.94,38.816,-14.46));
#36735=CARTESIAN_POINT('',(-23.94,38.816,-14.46));
#36736=CARTESIAN_POINT('Origin',(-20.75,38.816,-14.46));
#36737=CARTESIAN_POINT('Origin',(-23.79,38.966,-7.23));
#36738=CARTESIAN_POINT('',(-23.94,38.816,14.46));
#36739=CARTESIAN_POINT('',(-23.94,38.816,14.46));
#36740=CARTESIAN_POINT('',(-23.94,38.816,-7.23));
#36741=CARTESIAN_POINT('Origin',(-20.75,38.966,14.46));
#36742=CARTESIAN_POINT('',(-20.75,38.816,17.65));
#36743=CARTESIAN_POINT('',(-20.75,38.816,17.65));
#36744=CARTESIAN_POINT('Origin',(-20.75,38.816,14.46));
#36745=CARTESIAN_POINT('Origin',(-2.535,38.966,17.5));
#36746=CARTESIAN_POINT('',(-2.535,38.816,17.65));
#36747=CARTESIAN_POINT('Origin',(17.13,38.966,10.73));
#36748=CARTESIAN_POINT('',(17.28,38.816,21.46));
#36749=CARTESIAN_POINT('',(17.28,38.816,10.73));
#36750=CARTESIAN_POINT('',(16.98,39.116,21.16));
#36751=CARTESIAN_POINT('Origin',(12.67,38.966,21.31));
#36752=CARTESIAN_POINT('',(9.66,38.816,21.46));
#36753=CARTESIAN_POINT('',(12.67,38.816,21.46));
#36754=CARTESIAN_POINT('',(9.96,39.116,21.16));
#36755=CARTESIAN_POINT('Origin',(9.81,38.966,8.5));
#36756=CARTESIAN_POINT('',(9.66,38.816,8.5));
#36757=CARTESIAN_POINT('Origin',(-17.28,35.936,-21.46));
#36758=CARTESIAN_POINT('',(-17.28,35.936,-21.46));
#36759=CARTESIAN_POINT('',(-17.28,35.936,-17.65));
#36760=CARTESIAN_POINT('Origin',(-9.66,35.936,-21.46));
#36761=CARTESIAN_POINT('',(-9.66,35.936,-21.46));
#36762=CARTESIAN_POINT('Origin',(-9.66,35.936,-17.));
#36763=CARTESIAN_POINT('',(-9.66,35.936,-17.65));
#36764=CARTESIAN_POINT('Origin',(52.11,35.936,-17.65));
#36765=CARTESIAN_POINT('',(9.66,35.936,-17.65));
#36766=CARTESIAN_POINT('Origin',(9.66,35.936,-21.46));
#36767=CARTESIAN_POINT('',(9.66,35.936,-21.46));
#36768=CARTESIAN_POINT('Origin',(17.28,35.936,-21.46));
#36769=CARTESIAN_POINT('',(17.28,35.936,-21.46));
#36770=CARTESIAN_POINT('Origin',(17.28,35.936,-17.));
#36771=CARTESIAN_POINT('',(17.28,35.936,-17.65));
#36772=CARTESIAN_POINT('Origin',(52.11,35.936,-17.65));
#36773=CARTESIAN_POINT('',(52.11,35.936,-17.65));
#36774=CARTESIAN_POINT('Origin',(52.11,35.936,-14.46));
#36775=CARTESIAN_POINT('',(55.3,35.936,-14.46));
#36776=CARTESIAN_POINT('Origin',(55.3,35.936,14.46));
#36777=CARTESIAN_POINT('',(55.3,35.936,14.46));
#36778=CARTESIAN_POINT('Origin',(52.11,35.936,14.46));
#36779=CARTESIAN_POINT('',(52.11,35.936,17.65));
#36780=CARTESIAN_POINT('Origin',(-20.75,35.936,17.65));
#36781=CARTESIAN_POINT('',(17.28,35.936,17.65));
#36782=CARTESIAN_POINT('Origin',(-1.305,38.966,2.625));
#36783=CARTESIAN_POINT('',(-14.16,38.816,2.475));
#36784=CARTESIAN_POINT('',(-18.29,38.816,2.475));
#36785=CARTESIAN_POINT('',(-1.305,38.816,2.475));
#36786=CARTESIAN_POINT('',(-18.29,38.816,2.475));
#36787=CARTESIAN_POINT('',(-14.46,39.116,2.775));
#36788=CARTESIAN_POINT('Origin',(45.67,38.966,6.84));
#36789=CARTESIAN_POINT('',(45.52,38.816,2.475));
#36790=CARTESIAN_POINT('',(45.52,38.816,13.68));
#36791=CARTESIAN_POINT('',(45.52,38.816,6.84));
#36792=CARTESIAN_POINT('',(45.52,38.816,13.68));
#36793=CARTESIAN_POINT('',(45.82,39.116,2.775));
#36794=CARTESIAN_POINT('Origin',(32.665,38.966,-2.625));
#36795=CARTESIAN_POINT('',(45.52,38.816,-2.475));
#36796=CARTESIAN_POINT('',(49.65,38.816,-2.475));
#36797=CARTESIAN_POINT('',(32.665,38.816,-2.475));
#36798=CARTESIAN_POINT('',(49.65,38.816,-2.475));
#36799=CARTESIAN_POINT('',(45.82,39.116,-2.775));
#36800=CARTESIAN_POINT('Origin',(49.65,38.966,0.));
#36801=CARTESIAN_POINT('',(49.65,38.816,2.475));
#36802=CARTESIAN_POINT('',(49.65,38.816,2.475));
#36803=CARTESIAN_POINT('Origin',(49.65,38.816,0.));
#36804=CARTESIAN_POINT('Origin',(30.595,38.966,2.625));
#36805=CARTESIAN_POINT('',(30.595,38.816,2.475));
#36806=CARTESIAN_POINT('Origin',(-14.31,38.966,-6.84));
#36807=CARTESIAN_POINT('',(-14.16,38.816,-2.475));
#36808=CARTESIAN_POINT('',(-14.16,38.816,-13.68));
#36809=CARTESIAN_POINT('',(-14.16,38.816,-6.84));
#36810=CARTESIAN_POINT('',(-14.16,38.816,-13.68));
#36811=CARTESIAN_POINT('',(-14.46,39.116,-2.775));
#36812=CARTESIAN_POINT('Origin',(-13.36,38.966,-13.68));
#36813=CARTESIAN_POINT('',(-13.36,38.816,-14.48));
#36814=CARTESIAN_POINT('',(-13.36,38.816,-14.48));
#36815=CARTESIAN_POINT('Origin',(-13.36,38.816,-13.68));
#36816=CARTESIAN_POINT('Origin',(30.2,38.966,-14.63));
#36817=CARTESIAN_POINT('',(44.72,38.816,-14.48));
#36818=CARTESIAN_POINT('',(44.72,38.816,-14.48));
#36819=CARTESIAN_POINT('',(30.2,38.816,-14.48));
#36820=CARTESIAN_POINT('Origin',(44.72,38.966,-13.68));
#36821=CARTESIAN_POINT('',(45.52,38.816,-13.68));
#36822=CARTESIAN_POINT('',(45.52,38.816,-13.68));
#36823=CARTESIAN_POINT('Origin',(44.72,38.816,-13.68));
#36824=CARTESIAN_POINT('Origin',(45.67,38.966,6.84));
#36825=CARTESIAN_POINT('',(45.52,38.816,6.84));
#36826=CARTESIAN_POINT('Origin',(44.72,38.966,13.68));
#36827=CARTESIAN_POINT('',(44.72,38.816,14.48));
#36828=CARTESIAN_POINT('',(44.72,38.816,14.48));
#36829=CARTESIAN_POINT('Origin',(44.72,38.816,13.68));
#36830=CARTESIAN_POINT('Origin',(1.16,38.966,14.63));
#36831=CARTESIAN_POINT('',(-13.36,38.816,14.48));
#36832=CARTESIAN_POINT('',(-13.36,38.816,14.48));
#36833=CARTESIAN_POINT('',(1.16,38.816,14.48));
#36834=CARTESIAN_POINT('Origin',(-13.36,38.966,13.68));
#36835=CARTESIAN_POINT('',(-14.16,38.816,13.68));
#36836=CARTESIAN_POINT('',(-14.16,38.816,13.68));
#36837=CARTESIAN_POINT('Origin',(-13.36,38.816,13.68));
#36838=CARTESIAN_POINT('Origin',(-14.31,38.966,-6.84));
#36839=CARTESIAN_POINT('',(-14.16,38.816,-6.84));
#36840=CARTESIAN_POINT('Origin',(-18.29,38.966,0.));
#36841=CARTESIAN_POINT('',(-18.29,38.816,-2.475));
#36842=CARTESIAN_POINT('',(-18.29,38.816,-2.475));
#36843=CARTESIAN_POINT('Origin',(-18.29,38.816,0.));
#36844=CARTESIAN_POINT('Origin',(0.765,38.966,-2.625));
#36845=CARTESIAN_POINT('',(0.765,38.816,-2.475));
#36846=CARTESIAN_POINT('Origin',(45.51,35.936,2.475));
#36847=CARTESIAN_POINT('',(49.65,35.936,2.475));
#36848=CARTESIAN_POINT('',(45.52,35.936,2.475));
#36849=CARTESIAN_POINT('Origin',(49.65,35.936,0.));
#36850=CARTESIAN_POINT('',(49.65,35.936,-2.475));
#36851=CARTESIAN_POINT('Origin',(49.65,35.936,-2.475));
#36852=CARTESIAN_POINT('',(45.52,35.936,-2.475));
#36853=CARTESIAN_POINT('Origin',(45.52,35.936,13.68));
#36854=CARTESIAN_POINT('',(45.52,35.936,-13.68));
#36855=CARTESIAN_POINT('Origin',(44.72,35.936,-13.68));
#36856=CARTESIAN_POINT('',(44.72,35.936,-14.48));
#36857=CARTESIAN_POINT('Origin',(44.72,35.936,-14.48));
#36858=CARTESIAN_POINT('',(-13.36,35.936,-14.48));
#36859=CARTESIAN_POINT('Origin',(-13.36,35.936,-13.68));
#36860=CARTESIAN_POINT('',(-14.16,35.936,-13.68));
#36861=CARTESIAN_POINT('Origin',(-14.16,35.936,-13.68));
#36862=CARTESIAN_POINT('',(-14.16,35.936,-2.475));
#36863=CARTESIAN_POINT('Origin',(-14.15,35.936,-2.475));
#36864=CARTESIAN_POINT('',(-18.29,35.936,-2.475));
#36865=CARTESIAN_POINT('Origin',(-18.29,35.936,2.475));
#36866=CARTESIAN_POINT('',(-14.16,35.936,2.475));
#36867=CARTESIAN_POINT('',(-18.29,35.936,2.475));
#36868=CARTESIAN_POINT('Origin',(-18.29,35.936,0.));
#36869=CARTESIAN_POINT('Origin',(45.52,35.936,13.68));
#36870=CARTESIAN_POINT('',(45.52,35.936,13.68));
#36871=CARTESIAN_POINT('Origin',(-14.16,35.936,-13.68));
#36872=CARTESIAN_POINT('',(-14.16,35.936,13.68));
#36873=CARTESIAN_POINT('Origin',(44.72,35.936,13.68));
#36874=CARTESIAN_POINT('',(44.72,35.936,14.48));
#36875=CARTESIAN_POINT('Origin',(-13.36,35.936,14.48));
#36876=CARTESIAN_POINT('',(-13.36,35.936,14.48));
#36877=CARTESIAN_POINT('Origin',(-13.36,35.936,13.68));
#36878=CARTESIAN_POINT('Origin',(17.28,35.936,21.46));
#36879=CARTESIAN_POINT('',(17.28,35.936,21.46));
#36880=CARTESIAN_POINT('Origin',(9.66,35.936,17.));
#36881=CARTESIAN_POINT('',(9.66,35.936,17.65));
#36882=CARTESIAN_POINT('',(9.66,35.936,21.46));
#36883=CARTESIAN_POINT('Origin',(9.66,35.936,21.46));
#36884=CARTESIAN_POINT('Origin',(-20.75,35.936,17.65));
#36885=CARTESIAN_POINT('',(-9.66,35.936,17.65));
#36886=CARTESIAN_POINT('Origin',(-17.28,35.936,17.));
#36887=CARTESIAN_POINT('',(-17.28,35.936,17.65));
#36888=CARTESIAN_POINT('',(-17.28,35.936,21.46));
#36889=CARTESIAN_POINT('Origin',(-9.66,35.936,21.46));
#36890=CARTESIAN_POINT('',(-9.66,35.936,21.46));
#36891=CARTESIAN_POINT('Origin',(-17.28,35.936,21.46));
#36892=CARTESIAN_POINT('Origin',(-20.75,35.936,17.65));
#36893=CARTESIAN_POINT('',(-20.75,35.936,17.65));
#36894=CARTESIAN_POINT('Origin',(-20.75,35.936,14.46));
#36895=CARTESIAN_POINT('',(-23.94,35.936,14.46));
#36896=CARTESIAN_POINT('Origin',(-23.94,35.936,-14.46));
#36897=CARTESIAN_POINT('',(-23.94,35.936,-14.46));
#36898=CARTESIAN_POINT('Origin',(-20.75,35.936,-14.46));
#36899=CARTESIAN_POINT('',(-20.75,35.936,-17.65));
#36900=CARTESIAN_POINT('Origin',(52.11,35.936,-17.65));
#83190=UNCERTAINTY_MEASURE_WITH_UNIT(LENGTH_MEASURE(0.01),#83220,
'DISTANCE_ACCURACY_VALUE',
'Maximum model space distance between geometric entities at asserted c
onnectivities');
#83203=UNCERTAINTY_MEASURE_WITH_UNIT(LENGTH_MEASURE(0.01),#83220,
'DISTANCE_ACCURACY_VALUE',
'Maximum model space distance between geometric entities at asserted c
onnectivities');
#83206=(
GEOMETRIC_REPRESENTATION_CONTEXT(3)
GLOBAL_UNCERTAINTY_ASSIGNED_CONTEXT((#83190))
GLOBAL_UNIT_ASSIGNED_CONTEXT((#83220,#83222,#83223))
REPRESENTATION_CONTEXT('','3D')
);
#83219=(
GEOMETRIC_REPRESENTATION_CONTEXT(3)
GLOBAL_UNCERTAINTY_ASSIGNED_CONTEXT((#83203))
GLOBAL_UNIT_ASSIGNED_CONTEXT((#83220,#83222,#83223))
REPRESENTATION_CONTEXT('','3D')
);
#83220=(
LENGTH_UNIT()
NAMED_UNIT(*)
SI_UNIT(.MILLI.,.METRE.)
);
#83222=(
NAMED_UNIT(*)
PLANE_ANGLE_UNIT()
SI_UNIT($,.RADIAN.)
);
#83223=(
NAMED_UNIT(*)
SI_UNIT($,.STERADIAN.)
SOLID_ANGLE_UNIT()
);
#83226=SHAPE_DEFINITION_REPRESENTATION(#83241,#83301);
#83241=PRODUCT_DEFINITION_SHAPE('',$,#83317);
#83301=SHAPE_REPRESENTATION('',(#27207),#83206);
#83314=PRODUCT_DEFINITION_CONTEXT('part definition',#83361,'design');
#83317=PRODUCT_DEFINITION('Large Servo Plate A','Large Servo Plate A',#83332,
#83314);
#83332=PRODUCT_DEFINITION_FORMATION('',$,#83365);
#83361=APPLICATION_CONTEXT(
'Core Data for Automotive Mechanical Design Process');
#83362=PRODUCT_CONTEXT('part definition',#83361,'mechanical');
#83365=PRODUCT('Large Servo Plate A','Large Servo Plate A',$,(#83362));
#83380=PRESENTATION_STYLE_ASSIGNMENT((#83395));
#83395=SURFACE_STYLE_USAGE(.BOTH.,#83410);
#83410=SURFACE_SIDE_STYLE('',(#83425));
#83425=SURFACE_STYLE_FILL_AREA(#83440);
#83440=FILL_AREA_STYLE('Opaque(218,221,226)',(#83455));
#83455=FILL_AREA_STYLE_COLOUR('Opaque(218,221,226)',#83470);
#83470=COLOUR_RGB('Opaque(218,221,226)', 0.31764706, 0.68627451, 0.89019608);
ENDSEC;
END-ISO-10303-21;
